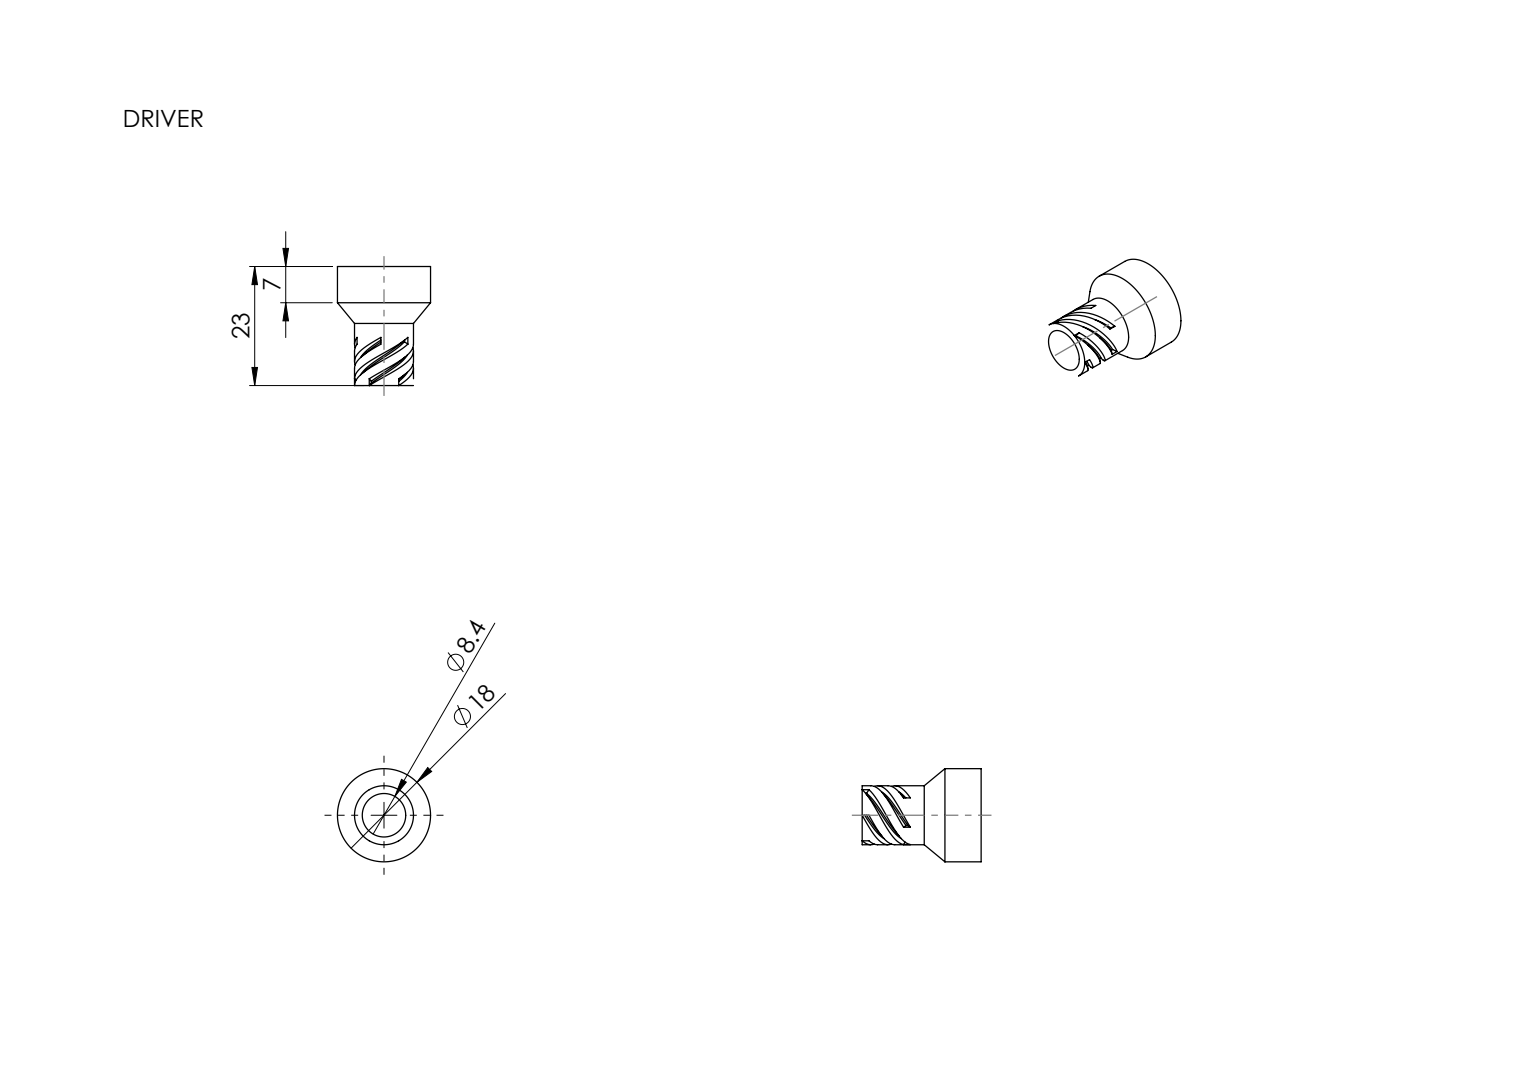
ISO-10303-21;
HEADER;
FILE_DESCRIPTION (('STEP AP214'),
    '1' );
FILE_NAME ('DRIVER.step',
    '2026-10-08T05:56:58',
    ( '' ),
    ( '' ),
    'SwSTEP 2.0',
    'SolidWorks 2026',
    '' );
FILE_SCHEMA (( 'AUTOMOTIVE_DESIGN' ));
ENDSEC;

DATA;
#10=ORIENTED_EDGE ( 'NONE', *, *, #9147, .T. ) ;
#12=CARTESIAN_POINT ( 'NONE',  ( 1.510506337161861223, 4.648860486681953397, -12.84374999795161543 ) ) ;
#32=( BOUNDED_CURVE ( )  B_SPLINE_CURVE ( 2, ( #2369, #8482, #14588, #875, #19172, #5461, #16578, #8772, #11868, #7343, #19367, #11771, #17980, #5752, #6052 ),
 .UNSPECIFIED., .F., .F. ) 
 B_SPLINE_CURVE_WITH_KNOTS ( ( 3, 2, 2, 2, 2, 2, 2, 3 ),
 ( 0.000000000000000000, 0.05000000000000000278, 0.1000000000000000056, 0.1499999999999999944, 0.2000000000000000111, 0.2500000000000000000, 0.2999999999999999889, 0.3333180920165871863 ),
 .UNSPECIFIED. ) 
 CURVE ( )  GEOMETRIC_REPRESENTATION_ITEM ( )  RATIONAL_B_SPLINE_CURVE ( ( 1.000000000000000000, 0.9876883405951377704, 1.000000000000000000, 0.9876883405951377704, 1.000000000000000000, 0.9876883405951377704, 1.000000000000000000, 0.9876883405951377704, 1.000000000000000000, 0.9876883405951377704, 1.000000000000000000, 0.9876883405951377704, 1.000000000000000000, 0.9917959799814384247, 0.9945256517182510247 ) ) 
 REPRESENTATION_ITEM ( '' )  );
#37=CARTESIAN_POINT ( 'NONE',  ( -5.207209108562804722, 2.318398865532109276, -15.31249999590322552 ) ) ;
#50=CARTESIAN_POINT ( 'NONE',  ( -1.493657965219562511, -5.574407415329147852, -9.812499995903225525 ) ) ;
#51=EDGE_CURVE ( 'NONE', #4769, #2089, #9336, .T. ) ;
#83=CARTESIAN_POINT ( 'NONE',  ( -4.620319390059805187, 1.773574444220790136, -11.34374999795161543 ) ) ;
#115=ORIENTED_EDGE ( 'NONE', *, *, #15621, .F. ) ;
#134=EDGE_CURVE ( 'NONE', #16351, #5756, #19323, .T. ) ;
#154=CARTESIAN_POINT ( 'NONE',  ( -5.700000000000001066, -0.5990941410143296730, -13.64430100820692537 ) ) ;
#159=CARTESIAN_POINT ( 'NONE',  ( 4.465502636338025688, -1.988169868018592412, -14.84374999795161543 ) ) ;
#163=EDGE_CURVE ( 'NONE', #5395, #4220, #13751, .T. ) ;
#168=FACE_OUTER_BOUND ( 'NONE', #5426, .T. ) ;
#169=CARTESIAN_POINT ( 'NONE',  ( 5.421022142882364392, -1.761396867937238486, -8.312499995903225525 ) ) ;
#180=CARTESIAN_POINT ( 'NONE',  ( -5.387740456496247887, -2.068159791354146293, -12.81249999590322552 ) ) ;
#184=CARTESIAN_POINT ( 'NONE',  ( 2.246813503491833508, 4.409619785863906571, -12.96874999795161543 ) ) ;
#214=CARTESIAN_POINT ( 'NONE',  ( 3.954556930911861112, 2.873153789725825913, -14.84374999795161543 ) ) ;
#216=EDGE_CURVE ( 'NONE', #1617, #5986, #4540, .T. ) ;
#221=CARTESIAN_POINT ( 'NONE',  ( -4.888101187500000222, 0.7741991708318887166, -6.968749997951614539 ) ) ;
#230=CARTESIAN_POINT ( 'NONE',  ( -3.270778111535363131, -3.632567103900500971, -10.84374999795161543 ) ) ;
#231=CARTESIAN_POINT ( 'NONE',  ( 2.444050593750020095, 4.233219804643871598, -6.468749997951615427 ) ) ;
#232=CARTESIAN_POINT ( 'NONE',  ( 4.942249507334556036, -0.2590123213421313686, -9.968749997951617203 ) ) ;
#234=CARTESIAN_POINT ( 'NONE',  ( 4.200000000000000178, 0.000000000000000000, -28.99999999999999645 ) ) ;
#256=CARTESIAN_POINT ( 'NONE',  ( 2.318398865532073749, 5.207209108562820710, -10.31249999590322552 ) ) ;
#266=EDGE_LOOP ( 'NONE', ( #427, #17181, #9017, #11698, #10341, #16603 ) ) ;
#270=EDGE_LOOP ( 'NONE', ( #16817, #14274, #8811, #901, #1434 ) ) ;
#274=CARTESIAN_POINT ( 'NONE',  ( -4.936344801571327601, -2.849999999999954792, -12.31249999590322552 ) ) ;
#275=CARTESIAN_POINT ( 'NONE',  ( -5.668774803599153422, 0.5958122406256767256, -13.00000000000000533 ) ) ;
#278=CARTESIAN_POINT ( 'NONE',  ( -4.409619785863906571, 2.246813503491833508, -7.968749997951616315 ) ) ;
#306=CARTESIAN_POINT ( 'NONE',  ( -2.246813503491833508, 4.409619785863906571, -10.34374999795161543 ) ) ;
#328=CARTESIAN_POINT ( 'NONE',  ( 4.465502636338039011, 1.988169868018562436, -8.468749997951615427 ) ) ;
#329=CARTESIAN_POINT ( 'NONE',  ( 4.780397808154266848, 1.280903732194421218, -8.968749997951611874 ) ) ;
#334=VECTOR ( 'NONE', #14992, 1000.000000000000000 ) ;
#347=ORIENTED_EDGE ( 'NONE', *, *, #1908, .F. ) ;
#353=EDGE_CURVE ( 'NONE', #3827, #6550, #12668, .T. ) ;
#354=CARTESIAN_POINT ( 'NONE',  ( -3.270778111535288080, 3.632567103900569361, -12.84374999795161543 ) ) ;
#356=AXIS2_PLACEMENT_3D ( 'NONE', #1344, #12254, #12353 ) ;
#369=CARTESIAN_POINT ( 'NONE',  ( 0.3020334839682081163, -5.763142191869158992, -8.812499995903225525 ) ) ;
#373=CARTESIAN_POINT ( 'NONE',  ( -4.611396867937201272, 3.350375938067097437, -8.000000000000005329 ) ) ;
#386=CARTESIAN_POINT ( 'NONE',  ( 5.668774803599163192, 0.5958122406255991210, -9.000000000000005329 ) ) ;
#427=ORIENTED_EDGE ( 'NONE', *, *, #9117, .T. ) ;
#431=CARTESIAN_POINT ( 'NONE',  ( 4.447186883680864788, 3.231070400981779667, -14.11718749948790830 ) ) ;
#434=CARTESIAN_POINT ( 'NONE',  ( 4.620319390059819398, -1.773574444220757274, -10.96874999795161720 ) ) ;
#443=EDGE_CURVE ( 'NONE', #4220, #16711, #7630, .T. ) ;
#446=ORIENTED_EDGE ( 'NONE', *, *, #14016, .F. ) ;
#476=ADVANCED_FACE ( 'NONE', ( #8445 ), #15472, .T. ) ;
#480=CARTESIAN_POINT ( 'NONE',  ( -3.143139765844555900, 4.840010801796527318, -12.50000000000000533 ) ) ;
#488=VERTEX_POINT ( 'NONE', #13041 ) ;
#500=SURFACE_SIDE_STYLE ('',( #17201 ) ) ;
#502=DIRECTION ( 'NONE',  ( -0.000000000000000000, -0.000000000000000000, 1.000000000000000000 ) ) ;
#513=CARTESIAN_POINT ( 'NONE',  ( 5.668774803599156975, -0.5958122406256373127, -14.31249999590322552 ) ) ;
#529=CARTESIAN_POINT ( 'NONE',  ( -9.000000000000001776, 0.000000000000000000, -22.00000000000000000 ) ) ;
#532=CARTESIAN_POINT ( 'NONE',  ( 5.700000000000001954, -0.5990941410143687529, -10.98069898359950258 ) ) ;
#535=DIRECTION ( 'NONE',  ( 1.000000000000000000, 0.000000000000000000, 0.000000000000000000 ) ) ;
#537=CARTESIAN_POINT ( 'NONE',  ( -4.942249507334558700, -0.2590123213420631454, -13.34374999795161365 ) ) ;
#544=EDGE_LOOP ( 'NONE', ( #8721, #12859, #15196, #3818, #16637 ) ) ;
#571=CARTESIAN_POINT ( 'NONE',  ( -2.318398865532109721, -5.207209108562803834, -9.000000000000005329 ) ) ;
#575=ORIENTED_EDGE ( 'NONE', *, *, #10908, .T. ) ;
#595=CARTESIAN_POINT ( 'NONE',  ( -1.510506337161893642, -4.648860486681943627, -12.46874999795161543 ) ) ;
#598=CARTESIAN_POINT ( 'NONE',  ( 0.000000000000000000, 0.000000000000000000, -28.99999999999999645 ) ) ;
#604=CARTESIAN_POINT ( 'NONE',  ( 3.270778111535314281, -3.632567103900546712, -12.84374999795161543 ) ) ;
#615=EDGE_CURVE ( 'NONE', #13431, #17330, #7505, .T. ) ;
#631=EDGE_CURVE ( 'NONE', #9247, #8012, #19426, .T. ) ;
#634=CARTESIAN_POINT ( 'NONE',  ( 3.632567103900546712, 3.270778111535313837, -7.843749997951614539 ) ) ;
#645=CIRCLE ( 'NONE', #13735, 5.700000000000002842 ) ;
#647=CARTESIAN_POINT ( 'NONE',  ( 2.246813503491803310, -4.409619785863921670, -9.968749997951615427 ) ) ;
#652=EDGE_LOOP ( 'NONE', ( #11686, #13562, #787, #7989 ) ) ;
#678=CARTESIAN_POINT ( 'NONE',  ( -1.493657965219446382, 5.574407415329178939, -13.50000000000000533 ) ) ;
#684=( BOUNDED_CURVE ( )  B_SPLINE_CURVE ( 2, ( #2775, #16596, #17896, #2575, #14700, #16400, #18096, #2876, #8691, #8990, #898, #990, #7068, #11693, #17798, #4094, #14800 ),
 .UNSPECIFIED., .F., .F. ) 
 B_SPLINE_CURVE_WITH_KNOTS ( ( 3, 2, 2, 2, 2, 2, 2, 2, 3 ),
 ( 0.000000000000000000, 0.05000000000000000971, 0.1000000000000000194, 0.1499999999999999944, 0.2000000000000000389, 0.2500000000000000000, 0.2999999999999999889, 0.3499999999999999223, 0.4000000000000000777 ),
 .UNSPECIFIED. ) 
 CURVE ( )  GEOMETRIC_REPRESENTATION_ITEM ( )  RATIONAL_B_SPLINE_CURVE ( ( 1.000000000000000000, 0.9876883405951377704, 1.000000000000000000, 0.9876883405951377704, 1.000000000000000000, 0.9876883405951377704, 1.000000000000000000, 0.9876883405951377704, 1.000000000000000000, 0.9876883405951377704, 1.000000000000000000, 0.9876883405951377704, 1.000000000000000000, 0.9876883405951377704, 1.000000000000000000, 0.9876883405951377704, 1.000000000000000000 ) ) 
 REPRESENTATION_ITEM ( '' )  );
#693=CARTESIAN_POINT ( 'NONE',  ( 5.142044285764733935, -2.620002426024580000, -7.500000000000005329 ) ) ;
#700=VECTOR ( 'NONE', #12818, 1000.000000000000000 ) ;
#707=CARTESIAN_POINT ( 'NONE',  ( 3.954556930911861112, 2.873153789725825913, -14.84374999795161543 ) ) ;
#732=CARTESIAN_POINT ( 'NONE',  ( 4.611396867937200383, 3.350375938067097881, -15.31249999590322552 ) ) ;
#736=VERTEX_POINT ( 'NONE', #10923 ) ;
#745=CARTESIAN_POINT ( 'NONE',  ( 5.421022142882364392, -1.761396867937238486, -8.312499995903225525 ) ) ;
#757=CARTESIAN_POINT ( 'NONE',  ( 0.000000000000000000, 0.000000000000000000, -28.99999999999999645 ) ) ;
#760=B_SPLINE_CURVE_WITH_KNOTS ( 'NONE', 1,
 ( #6972, #5479 ),
 .UNSPECIFIED., .F., .F.,
 ( 2, 2 ),
 ( 0.000000000000000000, 1.000000000000000000 ),
 .UNSPECIFIED. ) ;
#768=VERTEX_POINT ( 'NONE', #1106 ) ;
#772=CARTESIAN_POINT ( 'NONE',  ( -4.780397808154273953, -1.280903732194386579, -8.968749997951611874 ) ) ;
#778=FACE_OUTER_BOUND ( 'NONE', #6078, .T. ) ;
#782=ORIENTED_EDGE ( 'NONE', *, *, #15988, .T. ) ;
#787=ORIENTED_EDGE ( 'NONE', *, *, #9672, .F. ) ;
#790=EDGE_CURVE ( 'NONE', #17079, #15015, #15922, .T. ) ;
#798=ORIENTED_EDGE ( 'NONE', *, *, #9859, .T. ) ;
#803=CARTESIAN_POINT ( 'NONE',  ( 1.493657965219485462, -5.574407415329169169, -14.81249999590322552 ) ) ;
#805=( BOUNDED_SURFACE ( )  B_SPLINE_SURFACE ( 1, 2, ( 
 ( #16231, #11437, #17538, #3824, #17827, #9121, #4217, #4316, #13231, #11820, #13517, #19717, #19317, #10427, #6000, #15122, #10232 ),
 ( #4119, #11722, #1314, #10524, #14925, #17927, #8719, #5609, #2806, #16728, #14826, #16326, #16528, #5906, #13620, #3008, #12123 ) ),
 .UNSPECIFIED., .F., .F., .F. ) 
 B_SPLINE_SURFACE_WITH_KNOTS ( ( 2, 2 ),
 ( 3, 2, 2, 2, 2, 2, 2, 2, 3 ),
 ( 0.000000000000000000, 1.000000000000000000 ),
 ( 0.000000000000000000, 0.05000000000000000278, 0.1000000000000000056, 0.1499999999999999944, 0.2000000000000000111, 0.2500000000000000000, 0.2999999999999999889, 0.3499999999999999778, 0.4000000000000000222 ),
 .UNSPECIFIED. ) 
 GEOMETRIC_REPRESENTATION_ITEM ( )  RATIONAL_B_SPLINE_SURFACE ( (
 ( 1.000000000000000000, 0.9876883405951377704, 1.000000000000000000, 0.9876883405951377704, 1.000000000000000000, 0.9876883405951377704, 1.000000000000000000, 0.9876883405951377704, 1.000000000000000000, 0.9876883405951377704, 1.000000000000000000, 0.9876883405951377704, 1.000000000000000000, 0.9876883405951377704, 1.000000000000000000, 0.9876883405951377704, 1.000000000000000000),
 ( 1.000000000000000000, 0.9876883405951377704, 1.000000000000000000, 0.9876883405951377704, 1.000000000000000000, 0.9876883405951377704, 1.000000000000000000, 0.9876883405951377704, 1.000000000000000000, 0.9876883405951377704, 1.000000000000000000, 0.9876883405951377704, 1.000000000000000000, 0.9876883405951377704, 1.000000000000000000, 0.9876883405951377704, 1.000000000000000000) ) ) 
 REPRESENTATION_ITEM ( '' )  SURFACE ( )  );
#838=EDGE_CURVE ( 'NONE', #8012, #12976, #9469, .T. ) ;
#842=CARTESIAN_POINT ( 'NONE',  ( 1.510506337161829027, -4.648860486681964055, -10.84374999795161543 ) ) ;
#847=VECTOR ( 'NONE', #4218, 1000.000000000000000 ) ;
#859=AXIS2_PLACEMENT_3D ( 'NONE', #9005, #17910, #4106 ) ;
#868=CARTESIAN_POINT ( 'NONE',  ( 4.861323657744406113, -0.5109457054261780096, -13.46874999795161543 ) ) ;
#875=CARTESIAN_POINT ( 'NONE',  ( -0.3020334839682475847, 5.763142191869157216, -7.500000000000005329 ) ) ;
#880=VECTOR ( 'NONE', #12534, 1000.000000000000000 ) ;
#896=CARTESIAN_POINT ( 'NONE',  ( 3.814044456245474279, -4.235925505221167064, -13.31249999590322730 ) ) ;
#898=CARTESIAN_POINT ( 'NONE',  ( 4.233219804643871598, -2.444050593750019651, -11.46874999795161543 ) ) ;
#901=ORIENTED_EDGE ( 'NONE', *, *, #9677, .T. ) ;
#903=CARTESIAN_POINT ( 'NONE',  ( -9.000000000000001776, 1.102182119232617911E-15, -22.00000000000000000 ) ) ;
#906=DIRECTION ( 'NONE',  ( 1.000000000000000000, 0.000000000000000000, 0.000000000000000000 ) ) ;
#909=CARTESIAN_POINT ( 'NONE',  ( -2.647025296874989664, 4.584782303107598267, -6.234374998975811266 ) ) ;
#915=DIRECTION ( 'NONE',  ( -0.000000000000000000, -0.000000000000000000, 1.000000000000000000 ) ) ;
#924=VECTOR ( 'NONE', #15469, 1000.000000000000000 ) ;
#947=CARTESIAN_POINT ( 'NONE',  ( -2.873153789725852558, -3.954556930911842016, -13.46874999795161543 ) ) ;
#958=CARTESIAN_POINT ( 'NONE',  ( -3.114526743279308896, -3.846120219227901149, -7.343749997951615427 ) ) ;
#959=FACE_OUTER_BOUND ( 'NONE', #270, .T. ) ;
#980=FACE_OUTER_BOUND ( 'NONE', #5717, .T. ) ;
#988=CARTESIAN_POINT ( 'NONE',  ( 4.465502636338039011, 1.988169868018562436, -8.843749997951615427 ) ) ;
#990=CARTESIAN_POINT ( 'NONE',  ( 3.846120219227923798, -3.114526743279282250, -11.96874999795161365 ) ) ;
#992=CARTESIAN_POINT ( 'NONE',  ( -3.270778111535363131, -3.632567103900500971, -10.84374999795161543 ) ) ;
#995=CARTESIAN_POINT ( 'NONE',  ( 4.235925505221166176, 3.814044456245473835, -8.312499995903225525 ) ) ;
#1012=CARTESIAN_POINT ( 'NONE',  ( -3.350375938067097437, 4.611396867937201272, -9.000000000000005329 ) ) ;
#1016=AXIS2_PLACEMENT_3D ( 'NONE', #3831, #10049, #2613 ) ;
#1022=CARTESIAN_POINT ( 'NONE',  ( -0.5958122406255597081, 5.668774803599165857, -14.00000000000000533 ) ) ;
#1025=CARTESIAN_POINT ( 'NONE',  ( 2.850000000000024070, 4.936344801571289409, -6.000000000000005329 ) ) ;
#1026=CARTESIAN_POINT ( 'NONE',  ( 5.699999596629369059, -0.002144393866035136480, -6.000593838912648081 ) ) ;
#1050=ORIENTED_EDGE ( 'NONE', *, *, #3700, .F. ) ;
#1059=CARTESIAN_POINT ( 'NONE',  ( -4.233219804643852946, 2.444050593750049405, -11.84374999795161365 ) ) ;
#1061=CARTESIAN_POINT ( 'NONE',  ( 2.695436003842732298, 4.150607464521791634, -9.968749997951617203 ) ) ;
#1063=ORIENTED_EDGE ( 'NONE', *, *, #9677, .F. ) ;
#1073=B_SPLINE_CURVE_WITH_KNOTS ( 'NONE', 1,
 ( #8978, #2969 ),
 .UNSPECIFIED., .F., .F.,
 ( 2, 2 ),
 ( 0.000000000000000000, 1.000000000000000000 ),
 .UNSPECIFIED. ) ;
#1093=CARTESIAN_POINT ( 'NONE',  ( -4.080749450109650844, 4.080749450109650844, -9.812499995903223748 ) ) ;
#1099=EDGE_LOOP ( 'NONE', ( #1954, #16438, #575, #16915 ) ) ;
#1103=EDGE_CURVE ( 'NONE', #13293, #13685, #7982, .T. ) ;
#1106=CARTESIAN_POINT ( 'NONE',  ( -5.700000000000002842, 0.000000000000000000, -18.00000000000000355 ) ) ;
#1119=CARTESIAN_POINT ( 'NONE',  ( 4.611396867937200383, 3.350375938067097881, -14.00000000000000533 ) ) ;
#1130=CARTESIAN_POINT ( 'NONE',  ( 4.840010801796506001, 3.143139765844590983, -7.500000000000005329 ) ) ;
#1144=CARTESIAN_POINT ( 'NONE',  ( -3.954556930911881096, -2.873153789725797935, -14.46874999795161720 ) ) ;
#1146=CARTESIAN_POINT ( 'NONE',  ( -4.465502636338010589, 1.988169868018623720, -14.84374999795161543 ) ) ;
#1147=EDGE_LOOP ( 'NONE', ( #4096, #3789, #12811, #6049 ) ) ;
#1153=ORIENTED_EDGE ( 'NONE', *, *, #6590, .T. ) ;
#1156=CARTESIAN_POINT ( 'NONE',  ( 0.000000000000000000, 0.000000000000000000, -6.000000000000005329 ) ) ;
#1158=CARTESIAN_POINT ( 'NONE',  ( 4.465502636338025688, -1.988169868018592856, -14.46874999795161720 ) ) ;
#1160=CARTESIAN_POINT ( 'NONE',  ( 0.5958122406256377568, 5.668774803599156975, -9.312499995903225525 ) ) ;
#1195=CARTESIAN_POINT ( 'NONE',  ( 0.5958122406255995651, -5.668774803599162304, -14.00000000000000533 ) ) ;
#1196=EDGE_LOOP ( 'NONE', ( #11214, #10475, #18129, #3079 ) ) ;
#1206=CARTESIAN_POINT ( 'NONE',  ( 4.888101187500000222, -3.413342815706642518E-14, -6.468749997951615427 ) ) ;
#1224=CARTESIAN_POINT ( 'NONE',  ( 4.620319390059829168, 1.773574444220725299, -11.96874999795161365 ) ) ;
#1235=CARTESIAN_POINT ( 'NONE',  ( -3.499494075959840078, -3.499494075959791672, -14.34374999795161365 ) ) ;
#1256=CARTESIAN_POINT ( 'NONE',  ( -0.3020334839682475847, 5.763142191869157216, -7.500000000000005329 ) ) ;
#1288=CARTESIAN_POINT ( 'NONE',  ( -4.840010801796527318, -3.143139765844555900, -8.812499995903225525 ) ) ;
#1291=CARTESIAN_POINT ( 'NONE',  ( -4.942249507334554259, 0.2590123213421660631, -9.968749997951615427 ) ) ;
#1308=FACE_OUTER_BOUND ( 'NONE', #10180, .T. ) ;
#1314=CARTESIAN_POINT ( 'NONE',  ( 1.016293382781377819, -4.781284448697200595, -7.468749997951615427 ) ) ;
#1320=CARTESIAN_POINT ( 'NONE',  ( -3.499494075959840078, -3.499494075959792116, -14.34374999795161543 ) ) ;
#1322=CARTESIAN_POINT ( 'NONE',  ( -0.2590123213420971182, 4.942249507334556924, -7.968749997951616315 ) ) ;
#1343=ORIENTED_EDGE ( 'NONE', *, *, #8950, .F. ) ;
#1344=CARTESIAN_POINT ( 'NONE',  ( 2.647025296875021638, 4.584782303107579615, -6.234374998975811266 ) ) ;
#1346=VERTEX_POINT ( 'NONE', #4276 ) ;
#1349=VECTOR ( 'NONE', #9495, 1000.000000000000000 ) ;
#1350=CARTESIAN_POINT ( 'NONE',  ( 1.988169868018562880, -4.465502636338038123, -13.46874999795161543 ) ) ;
#1358=CARTESIAN_POINT ( 'NONE',  ( 5.207209108562820710, -2.318398865532073305, -14.00000000000000533 ) ) ;
#1384=ORIENTED_EDGE ( 'NONE', *, *, #5542, .T. ) ;
#1389=CARTESIAN_POINT ( 'NONE',  ( -5.700000000000000178, 0.5990941410143899581, -9.668198987696271729 ) ) ;
#1392=CARTESIAN_POINT ( 'NONE',  ( 4.465502636338025688, -1.988169868018592412, -14.84374999795161543 ) ) ;
#1393=CARTESIAN_POINT ( 'NONE',  ( -5.387740456496206143, 2.068159791354259092, -11.81249999590322552 ) ) ;
#1396=CARTESIAN_POINT ( 'NONE',  ( -4.233219804643852946, 2.444050593750049405, -11.46874999795161543 ) ) ;
#1422=AXIS2_PLACEMENT_3D ( 'NONE', #9159, #13556, #15159 ) ;
#1423=CARTESIAN_POINT ( 'NONE',  ( -2.647025296874989664, 4.584782303107598267, -7.078124996927420476 ) ) ;
#1426=CARTESIAN_POINT ( 'NONE',  ( 4.233219804643887585, 2.444050593749990785, -11.46874999795161543 ) ) ;
#1434=ORIENTED_EDGE ( 'NONE', *, *, #14888, .F. ) ;
#1458=CARTESIAN_POINT ( 'NONE',  ( 4.484949146646379781, 3.631840208645794821, -10.50000000000000711 ) ) ;
#1462=VERTEX_POINT ( 'NONE', #14451 ) ;
#1474=CARTESIAN_POINT ( 'NONE',  ( 1.761396867937162769, -5.421022142882388373, -11.31249999590322375 ) ) ;
#1487=CARTESIAN_POINT ( 'NONE',  ( 0.7741991708318884946, 4.888101187500000222, -12.34374999795161543 ) ) ;
#1504=CARTESIAN_POINT ( 'NONE',  ( 1.988169868018562880, -4.465502636338038123, -13.84374999795161543 ) ) ;
#1514=VERTEX_POINT ( 'NONE', #9958 ) ;
#1524=CARTESIAN_POINT ( 'NONE',  ( -3.954556930911862000, 2.873153789725825469, -8.468749997951615427 ) ) ;
#1532=CARTESIAN_POINT ( 'NONE',  ( 5.294050593750000644, -3.696815770993907903E-14, -6.234374998975811266 ) ) ;
#1536=CARTESIAN_POINT ( 'NONE',  ( -5.668774803599165857, -0.5958122406255588199, -9.000000000000005329 ) ) ;
#1550=CARTESIAN_POINT ( 'NONE',  ( 2.850000000000024070, 4.936344801571289409, -6.000000000000005329 ) ) ;
#1554=CARTESIAN_POINT ( 'NONE',  ( -5.763142191869158992, -0.3020334839682081163, -12.50000000000000533 ) ) ;
#1556=ORIENTED_EDGE ( 'NONE', *, *, #8950, .T. ) ;
#1557=( BOUNDED_CURVE ( )  B_SPLINE_CURVE ( 2, ( #1026, #14552, #14649, #11354, #13044, #18945, #11448, #13241, #2522, #8631, #5527, #5429, #7110, #19233, #19328, #8541, #5235 ),
 .UNSPECIFIED., .F., .F. ) 
 B_SPLINE_CURVE_WITH_KNOTS ( ( 3, 2, 2, 2, 2, 2, 2, 2, 3 ),
 ( 0.000000000000000000, 0.05000000000000000971, 0.1000000000000000194, 0.1499999999999999944, 0.2000000000000000389, 0.2500000000000000000, 0.2999999999999999889, 0.3499999999999999223, 0.4000000000000000777 ),
 .UNSPECIFIED. ) 
 CURVE ( )  GEOMETRIC_REPRESENTATION_ITEM ( )  RATIONAL_B_SPLINE_CURVE ( ( 1.000000000000000000, 0.9876883405951377704, 1.000000000000000000, 0.9876883405951377704, 1.000000000000000000, 0.9876883405951377704, 1.000000000000000000, 0.9876883405951377704, 1.000000000000000000, 0.9876883405951377704, 1.000000000000000000, 0.9876883405951377704, 1.000000000000000000, 0.9876883405951377704, 1.000000000000000000, 0.9876883405951377704, 1.000000000000000000 ) ) 
 REPRESENTATION_ITEM ( '' )  );
#1609=VECTOR ( 'NONE', #17718, 1000.000000000000000 ) ;
#1615=CARTESIAN_POINT ( 'NONE',  ( -3.954556930911862000, 2.873153789725825469, -8.843749997951615427 ) ) ;
#1617=VERTEX_POINT ( 'NONE', #13630 ) ;
#1633=ORIENTED_EDGE ( 'NONE', *, *, #14674, .F. ) ;
#1653=CARTESIAN_POINT ( 'NONE',  ( -5.387740456496247887, -2.068159791354146293, -11.50000000000000355 ) ) ;
#1654=CARTESIAN_POINT ( 'NONE',  ( -5.700000000000000178, -2.180340287075187351E-16, -13.97977757194593273 ) ) ;
#1660=EDGE_CURVE ( 'NONE', #5242, #16351, #10502, .T. ) ;
#1670=( BOUNDED_CURVE ( )  B_SPLINE_CURVE ( 2, ( #7922, #19032, #5323, #12936, #2509, #11720, #1012, #17925, #7193, #4117, #6811, #19128, #8717, #14824, #17727, #7095, #1119 ),
 .UNSPECIFIED., .F., .F. ) 
 B_SPLINE_CURVE_WITH_KNOTS ( ( 3, 2, 2, 2, 2, 2, 2, 2, 3 ),
 ( 0.000000000000000000, 0.05000000000000000971, 0.1000000000000000194, 0.1499999999999999944, 0.2000000000000000389, 0.2500000000000000000, 0.2999999999999999889, 0.3499999999999999223, 0.4000000000000000777 ),
 .UNSPECIFIED. ) 
 CURVE ( )  GEOMETRIC_REPRESENTATION_ITEM ( )  RATIONAL_B_SPLINE_CURVE ( ( 1.000000000000000000, 0.9876883405951377704, 1.000000000000000000, 0.9876883405951377704, 1.000000000000000000, 0.9876883405951377704, 1.000000000000000000, 0.9876883405951377704, 1.000000000000000000, 0.9876883405951377704, 1.000000000000000000, 0.9876883405951377704, 1.000000000000000000, 0.9876883405951377704, 1.000000000000000000, 0.9876883405951377704, 1.000000000000000000 ) ) 
 REPRESENTATION_ITEM ( '' )  );
#1686=CARTESIAN_POINT ( 'NONE',  ( -1.988169868018530906, 4.465502636338051445, -13.84374999795161543 ) ) ;
#1692=DIRECTION ( 'NONE',  ( 0.4330127018922284576, 0.7499999999999961142, 0.4999999999999977240 ) ) ;
#1696=CARTESIAN_POINT ( 'NONE',  ( -5.668774803599165857, -0.5958122406255588199, -10.31249999590322552 ) ) ;
#1708=CARTESIAN_POINT ( 'NONE',  ( 1.493657965219485462, -5.574407415329169169, -13.50000000000000533 ) ) ;
#1714=CARTESIAN_POINT ( 'NONE',  ( -3.954556930911862000, 2.873153789725825469, -8.843749997951615427 ) ) ;
#1759=CARTESIAN_POINT ( 'NONE',  ( 5.763142191869157216, 0.3020334839682480288, -13.81249999590322552 ) ) ;
#1779=CARTESIAN_POINT ( 'NONE',  ( -1.761396867937200739, 5.421022142882375938, -10.00000000000000533 ) ) ;
#1791=CARTESIAN_POINT ( 'NONE',  ( -4.611396867937224364, -3.350375938067065906, -14.00000000000000533 ) ) ;
#1794=( NAMED_UNIT ( * ) SI_UNIT ( $, .STERADIAN. ) SOLID_ANGLE_UNIT ( ) );
#1808=EDGE_LOOP ( 'NONE', ( #15620, #13680, #16181, #1384 ) ) ;
#1810=FACE_OUTER_BOUND ( 'NONE', #1196, .T. ) ;
#1816=AXIS2_PLACEMENT_3D ( 'NONE', #1532, #10443, #7619 ) ;
#1820=VECTOR ( 'NONE', #5810, 1000.000000000000000 ) ;
#1821=ORIENTED_EDGE ( 'NONE', *, *, #10236, .T. ) ;
#1824=CARTESIAN_POINT ( 'NONE',  ( 5.700000000000002842, 2.725425358843983450E-16, -10.64522241986047568 ) ) ;
#1874=CARTESIAN_POINT ( 'NONE',  ( -3.143139765844656708, -4.840010801796461593, -10.81249999590322375 ) ) ;
#1877=CARTESIAN_POINT ( 'NONE',  ( -2.246813503491833508, 4.409619785863906571, -9.968749997951617203 ) ) ;
#1883=CARTESIAN_POINT ( 'NONE',  ( -2.647025296875054057, -4.584782303107560963, -7.078124996927420476 ) ) ;
#1888=CARTESIAN_POINT ( 'NONE',  ( -3.631840208645857437, -4.484949146646330931, -7.812499995903224637 ) ) ;
#1894=DIRECTION ( 'NONE',  ( 1.000000000000000000, 0.000000000000000000, 0.000000000000000000 ) ) ;
#1899=VERTEX_POINT ( 'NONE', #6993 ) ;
#1908=EDGE_CURVE ( 'NONE', #7839, #10504, #16759, .T. ) ;
#1914=ORIENTED_EDGE ( 'NONE', *, *, #9622, .T. ) ;
#1925=CARTESIAN_POINT ( 'NONE',  ( 4.861323657744411442, 0.5109457054261445919, -9.468749997951615427 ) ) ;
#1941=SHAPE_DEFINITION_REPRESENTATION ( #10190, #6040 ) ;
#1942=CARTESIAN_POINT ( 'NONE',  ( -3.143139765844656708, -4.840010801796461593, -9.500000000000003553 ) ) ;
#1954=ORIENTED_EDGE ( 'NONE', *, *, #9226, .T. ) ;
#1959=CARTESIAN_POINT ( 'NONE',  ( -5.387740456496247887, -2.068159791354146293, -11.50000000000000355 ) ) ;
#1971=CARTESIAN_POINT ( 'NONE',  ( -2.318398865532001363, 5.207209108562852684, -14.31249999590322552 ) ) ;
#1978=CARTESIAN_POINT ( 'NONE',  ( 5.207209108562820710, -2.318398865532073305, -14.00000000000000533 ) ) ;
#1985=CARTESIAN_POINT ( 'NONE',  ( -3.499494075959840078, -3.499494075959791672, -13.96874999795161365 ) ) ;
#1989=LINE ( 'NONE', #13905, #16458 ) ;
#1996=CARTESIAN_POINT ( 'NONE',  ( 5.700000000000002842, 2.725425358843983450E-16, -9.332722423957255486 ) ) ;
#2001=CARTESIAN_POINT ( 'NONE',  ( 5.207209108562820710, -2.318398865532073305, -15.31249999590322552 ) ) ;
#2013=ORIENTED_EDGE ( 'NONE', *, *, #9226, .F. ) ;
#2027=CARTESIAN_POINT ( 'NONE',  ( 4.781284448697187273, -1.016293382781444654, -10.46874999795161720 ) ) ;
#2031=CARTESIAN_POINT ( 'NONE',  ( 5.207209108562820710, -2.318398865532073305, -15.31249999590322552 ) ) ;
#2053=CARTESIAN_POINT ( 'NONE',  ( -4.861323657744413218, -0.5109457054261099529, -9.843749997951615427 ) ) ;
#2066=ORIENTED_EDGE ( 'NONE', *, *, #4858, .T. ) ;
#2072=CARTESIAN_POINT ( 'NONE',  ( -4.080749450109650844, 4.080749450109650844, -8.500000000000007105 ) ) ;
#2082=EDGE_CURVE ( 'NONE', #3194, #17426, #1989, .T. ) ;
#2083=CARTESIAN_POINT ( 'NONE',  ( 3.499494075959791672, -3.499494075959840966, -8.968749997951611874 ) ) ;
#2086=PRESENTATION_STYLE_ASSIGNMENT (( #5182 ) ) ;
#2089=VERTEX_POINT ( 'NONE', #9508 ) ;
#2093=CARTESIAN_POINT ( 'NONE',  ( 5.387740456496221242, -2.068159791354221344, -11.81249999590322552 ) ) ;
#2112=CARTESIAN_POINT ( 'NONE',  ( -5.700000000000000178, 0.5990941410143899581, -10.98069898359949192 ) ) ;
#2139=PLANE ( 'NONE',  #10424 ) ;
#2142=DIRECTION ( 'NONE',  ( 0.4330127018922234616, 0.7499999999999990008, 0.4999999999999978351 ) ) ;
#2154=CARTESIAN_POINT ( 'NONE',  ( -4.620319390059805187, 1.773574444220789914, -11.34374999795161543 ) ) ;
#2156=VECTOR ( 'NONE', #12013, 1000.000000000000000 ) ;
#2176=ORIENTED_EDGE ( 'NONE', *, *, #16459, .F. ) ;
#2179=EDGE_CURVE ( 'NONE', #8042, #9505, #19555, .T. ) ;
#2182=CARTESIAN_POINT ( 'NONE',  ( 2.246813503491803310, -4.409619785863921670, -9.968749997951617203 ) ) ;
#2189=CARTESIAN_POINT ( 'NONE',  ( 4.942249507334556036, -0.2590123213421313686, -10.34374999795161543 ) ) ;
#2190=( BOUNDED_CURVE ( )  B_SPLINE_CURVE ( 2, ( #18415, #15020, #19618, #13717, #2804, #7497, #6098, #18321, #5904, #12219, #10816, #15224, #12022, #16829, #10425, #18124, #2702 ),
 .UNSPECIFIED., .F., .F. ) 
 B_SPLINE_CURVE_WITH_KNOTS ( ( 3, 2, 2, 2, 2, 2, 2, 2, 3 ),
 ( 0.000000000000000000, 0.05000000000000000971, 0.1000000000000000194, 0.1499999999999999944, 0.2000000000000000389, 0.2500000000000000000, 0.2999999999999999889, 0.3499999999999999223, 0.4000000000000000777 ),
 .UNSPECIFIED. ) 
 CURVE ( )  GEOMETRIC_REPRESENTATION_ITEM ( )  RATIONAL_B_SPLINE_CURVE ( ( 1.000000000000000000, 0.9876883405951377704, 1.000000000000000000, 0.9876883405951377704, 1.000000000000000000, 0.9876883405951377704, 1.000000000000000000, 0.9876883405951377704, 1.000000000000000000, 0.9876883405951377704, 1.000000000000000000, 0.9876883405951377704, 1.000000000000000000, 0.9876883405951377704, 1.000000000000000000, 0.9876883405951377704, 1.000000000000000000 ) ) 
 REPRESENTATION_ITEM ( '' )  );
#2193=CARTESIAN_POINT ( 'NONE',  ( -2.873153789725825469, 3.954556930911862000, -9.843749997951615427 ) ) ;
#2194=EDGE_LOOP ( 'NONE', ( #16775, #7527, #12166, #10500 ) ) ;
#2196=ADVANCED_FACE ( 'NONE', ( #18598 ), #5183, .T. ) ;
#2201=FACE_OUTER_BOUND ( 'NONE', #18950, .T. ) ;
#2210=ORIENTED_EDGE ( 'NONE', *, *, #7191, .F. ) ;
#2218=CARTESIAN_POINT ( 'NONE',  ( 0.000000000000000000, 0.000000000000000000, -22.00000000000000000 ) ) ;
#2221=CARTESIAN_POINT ( 'NONE',  ( 3.632567103900546712, 3.270778111535313837, -7.468749997951615427 ) ) ;
#2222=ORIENTED_EDGE ( 'NONE', *, *, #15682, .F. ) ;
#2235=CARTESIAN_POINT ( 'NONE',  ( -1.510506337161893642, -4.648860486681943627, -12.46874999795161543 ) ) ;
#2261=EDGE_LOOP ( 'NONE', ( #7376, #6155, #6525, #11274, #6937 ) ) ;
#2317=CARTESIAN_POINT ( 'NONE',  ( 4.080749450109649956, 4.080749450109650844, -14.81249999590322375 ) ) ;
#2322=EDGE_CURVE ( 'NONE', #1899, #15854, #8394, .T. ) ;
#2330=CARTESIAN_POINT ( 'NONE',  ( 2.873153789725797491, -3.954556930911881985, -9.843749997951615427 ) ) ;
#2366=CARTESIAN_POINT ( 'NONE',  ( -4.611396867937224364, -3.350375938067065906, -15.31249999590322552 ) ) ;
#2369=CARTESIAN_POINT ( 'NONE',  ( -2.849999999999988987, 4.936344801571308061, -6.000000000000005329 ) ) ;
#2388=CARTESIAN_POINT ( 'NONE',  ( 3.632567103900546712, 3.270778111535313837, -7.843749997951614539 ) ) ;
#2391=CARTESIAN_POINT ( 'NONE',  ( 3.350375938067096548, 4.611396867937201272, -14.31249999590322552 ) ) ;
#2394=CARTESIAN_POINT ( 'NONE',  ( 5.207209108562838473, 2.318398865532038666, -9.312499995903225525 ) ) ;
#2400=FACE_OUTER_BOUND ( 'NONE', #5133, .T. ) ;
#2424=CARTESIAN_POINT ( 'NONE',  ( 0.5109457054261454800, -4.861323657744410554, -14.84374999795161543 ) ) ;
#2447=CARTESIAN_POINT ( 'NONE',  ( -4.942249507334553371, 0.2590123213421660631, -9.968749997951617203 ) ) ;
#2455=CARTESIAN_POINT ( 'NONE',  ( -4.781284448697179279, 1.016293382781477961, -10.46874999795161720 ) ) ;
#2478=CARTESIAN_POINT ( 'NONE',  ( 4.233219804643871598, -2.444050593750019651, -11.84374999795161365 ) ) ;
#2482=CARTESIAN_POINT ( 'NONE',  ( -0.9027913098498572264, 5.699999999999999289, -11.81249999590322552 ) ) ;
#2494=ORIENTED_EDGE ( 'NONE', *, *, #10561, .T. ) ;
#2496=CARTESIAN_POINT ( 'NONE',  ( 3.954556930911861112, 2.873153789725825913, -14.46874999795161720 ) ) ;
#2509=CARTESIAN_POINT ( 'NONE',  ( -4.611396867937201272, 3.350375938067097437, -8.000000000000005329 ) ) ;
#2517=CARTESIAN_POINT ( 'NONE',  ( -0.5109457054261112852, 4.861323657744413218, -14.46874999795161720 ) ) ;
#2522=CARTESIAN_POINT ( 'NONE',  ( 1.761396867937162769, -5.421022142882388373, -10.00000000000000533 ) ) ;
#2540=DIRECTION ( 'NONE',  ( 1.000000000000000000, 0.000000000000000000, 0.000000000000000000 ) ) ;
#2544=CARTESIAN_POINT ( 'NONE',  ( -2.444050593749990341, 4.233219804643887585, -6.468749997951615427 ) ) ;
#2574=CARTESIAN_POINT ( 'NONE',  ( -2.318398865532001363, 5.207209108562852684, -13.00000000000000533 ) ) ;
#2575=CARTESIAN_POINT ( 'NONE',  ( 4.150607464521811174, 2.695436003842704764, -7.968749997951616315 ) ) ;
#2577=CARTESIAN_POINT ( 'NONE',  ( 0.9027913098498566713, 5.699999999999999289, -12.81249999590322552 ) ) ;
#2582=CARTESIAN_POINT ( 'NONE',  ( 5.700000000000001954, 0.2987243419133224775, -10.47794484381774538 ) ) ;
#2597=VERTEX_POINT ( 'NONE', #12384 ) ;
#2603=CARTESIAN_POINT ( 'NONE',  ( -1.761396867937200739, 5.421022142882375938, -11.31249999590322375 ) ) ;
#2613=DIRECTION ( 'NONE',  ( 1.000000000000000000, 0.000000000000000000, 0.000000000000000000 ) ) ;
#2616=CARTESIAN_POINT ( 'NONE',  ( 1.280903732194454303, 4.780397808154257078, -8.968749997951611874 ) ) ;
#2642=DIRECTION ( 'NONE',  ( -0.000000000000000000, -0.000000000000000000, 1.000000000000000000 ) ) ;
#2643=VECTOR ( 'NONE', #18602, 1000.000000000000000 ) ;
#2645=VERTEX_POINT ( 'NONE', #8564 ) ;
#2658=VECTOR ( 'NONE', #17100, 1000.000000000000114 ) ;
#2672=LINE ( 'NONE', #8788, #16879 ) ;
#2674=CARTESIAN_POINT ( 'NONE',  ( -5.387740456496205255, 2.068159791354258648, -10.50000000000000533 ) ) ;
#2680=CARTESIAN_POINT ( 'NONE',  ( 5.668774803599163192, 0.5958122406255991210, -10.31249999590322552 ) ) ;
#2684=EDGE_CURVE ( 'NONE', #12845, #19252, #3862, .T. ) ;
#2692=CARTESIAN_POINT ( 'NONE',  ( 3.846120219227923798, -3.114526743279282250, -12.34374999795161543 ) ) ;
#2695=ADVANCED_FACE ( 'NONE', ( #959 ), #16118, .T. ) ;
#2702=CARTESIAN_POINT ( 'NONE',  ( 4.465502636338025688, -1.988169868018592412, -14.84374999795161543 ) ) ;
#2711=ADVANCED_FACE ( 'NONE', ( #7138 ), #14866, .F. ) ;
#2713=CARTESIAN_POINT ( 'NONE',  ( -3.383411828340740850E-14, -4.888101187500000222, -11.84374999795161365 ) ) ;
#2715=CARTESIAN_POINT ( 'NONE',  ( 0.5109457054261784537, 4.861323657744407001, -8.843749997951615427 ) ) ;
#2718=ORIENTED_EDGE ( 'NONE', *, *, #18316, .F. ) ;
#2740=CARTESIAN_POINT ( 'NONE',  ( 4.942249507334556036, -0.2590123213421313686, -9.968749997951617203 ) ) ;
#2746=CARTESIAN_POINT ( 'NONE',  ( 1.493657965219523875, 5.574407415329156734, -8.500000000000007105 ) ) ;
#2754=ADVANCED_FACE ( 'NONE', ( #16773 ), #12549, .T. ) ;
#2765=CARTESIAN_POINT ( 'NONE',  ( 5.142044285764733935, -2.620002426024580000, -8.812499995903225525 ) ) ;
#2768=DIRECTION ( 'NONE',  ( 1.000000000000000000, 0.000000000000000000, 0.000000000000000000 ) ) ;
#2774=LINE ( 'NONE', #8890, #334 ) ;
#2775=CARTESIAN_POINT ( 'NONE',  ( 2.444050593750020095, 4.233219804643871598, -6.468749997951615427 ) ) ;
#2781=CARTESIAN_POINT ( 'NONE',  ( -4.150607464521828938, -2.695436003842674122, -7.968749997951616315 ) ) ;
#2804=CARTESIAN_POINT ( 'NONE',  ( 0.5109457054261780096, 4.861323657744407001, -8.843749997951615427 ) ) ;
#2806=CARTESIAN_POINT ( 'NONE',  ( -3.270778111535363131, -3.632567103900500971, -10.46874999795161720 ) ) ;
#2811=CARTESIAN_POINT ( 'NONE',  ( -4.409619785863906571, 2.246813503491833508, -7.968749997951616315 ) ) ;
#2830=CARTESIAN_POINT ( 'NONE',  ( -3.954556930911881096, -2.873153789725797935, -14.84374999795161543 ) ) ;
#2831=( BOUNDED_CURVE ( )  B_SPLINE_CURVE ( 2, ( #15093, #1389, #4092, #2674, #7468, #7362, #16297, #4287, #2574, #7166, #19386 ),
 .UNSPECIFIED., .F., .F. ) 
 B_SPLINE_CURVE_WITH_KNOTS ( ( 3, 2, 2, 2, 2, 3 ),
 ( 0.1666819079834106210, 0.2000000000000000111, 0.2500000000000000000, 0.2999999999999999889, 0.3499999999999999778, 0.4000000000000000222 ),
 .UNSPECIFIED. ) 
 CURVE ( )  GEOMETRIC_REPRESENTATION_ITEM ( )  RATIONAL_B_SPLINE_CURVE ( ( 0.9945256517182514688, 0.9917959799814378696, 1.000000000000000000, 0.9876883405951377704, 1.000000000000000000, 0.9876883405951377704, 1.000000000000000000, 0.9876883405951377704, 1.000000000000000000, 0.9876883405951377704, 1.000000000000000000 ) ) 
 REPRESENTATION_ITEM ( '' )  );
#2840=ORIENTED_EDGE ( 'NONE', *, *, #9859, .F. ) ;
#2842=CARTESIAN_POINT ( 'NONE',  ( 3.143139765844590983, -4.840010801796506890, -12.50000000000000533 ) ) ;
#2848=CARTESIAN_POINT ( 'NONE',  ( 1.185096637661176677, -5.575441324182703440, -7.000000000000005329 ) ) ;
#2851=LINE ( 'NONE', #13565, #19746 ) ;
#2853=CARTESIAN_POINT ( 'NONE',  ( 3.814044456245502701, 4.235925505221138643, -11.31249999590322375 ) ) ;
#2875=LINE ( 'NONE', #5771, #17263 ) ;
#2876=CARTESIAN_POINT ( 'NONE',  ( 4.942249507334556036, -0.2590123213421313686, -9.968749997951615427 ) ) ;
#2877=CARTESIAN_POINT ( 'NONE',  ( -5.763142191869152775, 0.3020334839683282979, -10.81249999590322375 ) ) ;
#2880=DIRECTION ( 'NONE',  ( 1.000000000000000000, 0.000000000000000000, 0.000000000000000000 ) ) ;
#2893=CARTESIAN_POINT ( 'NONE',  ( -0.5958122406255597081, 5.668774803599165857, -15.31249999590322552 ) ) ;
#2910=CARTESIAN_POINT ( 'NONE',  ( -1.773574444220725077, 4.620319390059829168, -6.968749997951614539 ) ) ;
#2919=CARTESIAN_POINT ( 'NONE',  ( 3.954556930911861112, 2.873153789725825913, -14.46874999795161720 ) ) ;
#2922=CARTESIAN_POINT ( 'NONE',  ( 2.647025296875021638, 4.584782303107579615, -7.078124996927420476 ) ) ;
#2930=DIRECTION ( 'NONE',  ( 0.8090169943749512260, 0.5877852522924679191, 0.000000000000000000 ) ) ;
#2948=CARTESIAN_POINT ( 'NONE',  ( -3.814044456245531567, -4.235925505221111997, -11.31249999590322375 ) ) ;
#2950=( BOUNDED_SURFACE ( )  B_SPLINE_SURFACE ( 1, 2, ( 
 ( #15739, #9748, #634, #9848, #12833, #6408, #4932, #15838, #14035, #5026, #14335, #6709, #11036, #11340, #17439, #15938, #9542 ),
 ( #15543, #15639, #2221, #13940, #8018, #329, #1925, #232, #2027, #434, #6511, #12640, #10939, #17044, #11137, #6316, #3333 ) ),
 .UNSPECIFIED., .F., .F., .F. ) 
 B_SPLINE_SURFACE_WITH_KNOTS ( ( 2, 2 ),
 ( 3, 2, 2, 2, 2, 2, 2, 2, 3 ),
 ( 0.000000000000000000, 1.000000000000000000 ),
 ( 0.000000000000000000, 0.05000000000000000278, 0.1000000000000000056, 0.1499999999999999944, 0.2000000000000000111, 0.2500000000000000000, 0.2999999999999999889, 0.3499999999999999778, 0.4000000000000000222 ),
 .UNSPECIFIED. ) 
 GEOMETRIC_REPRESENTATION_ITEM ( )  RATIONAL_B_SPLINE_SURFACE ( (
 ( 1.000000000000000000, 0.9876883405951377704, 1.000000000000000000, 0.9876883405951377704, 1.000000000000000000, 0.9876883405951377704, 1.000000000000000000, 0.9876883405951377704, 1.000000000000000000, 0.9876883405951377704, 1.000000000000000000, 0.9876883405951377704, 1.000000000000000000, 0.9876883405951377704, 1.000000000000000000, 0.9876883405951377704, 1.000000000000000000),
 ( 1.000000000000000000, 0.9876883405951377704, 1.000000000000000000, 0.9876883405951377704, 1.000000000000000000, 0.9876883405951377704, 1.000000000000000000, 0.9876883405951377704, 1.000000000000000000, 0.9876883405951377704, 1.000000000000000000, 0.9876883405951377704, 1.000000000000000000, 0.9876883405951377704, 1.000000000000000000, 0.9876883405951377704, 1.000000000000000000) ) ) 
 REPRESENTATION_ITEM ( '' )  SURFACE ( )  );
#2969=CARTESIAN_POINT ( 'NONE',  ( -0.5109457054261112852, 4.861323657744413218, -14.84374999795161543 ) ) ;
#2981=CARTESIAN_POINT ( 'NONE',  ( 2.873153789725825025, 3.954556930911862000, -13.84374999795161543 ) ) ;
#3008=CARTESIAN_POINT ( 'NONE',  ( -4.780397808154247308, 1.280903732194486722, -13.96874999795161365 ) ) ;
#3014=CARTESIAN_POINT ( 'NONE',  ( 2.873153789725797491, -3.954556930911881985, -9.843749997951615427 ) ) ;
#3015=ORIENTED_EDGE ( 'NONE', *, *, #12236, .T. ) ;
#3017=CARTESIAN_POINT ( 'NONE',  ( -2.873153789725825469, 3.954556930911862000, -9.468749997951615427 ) ) ;
#3022=EDGE_LOOP ( 'NONE', ( #7553, #18998, #8944, #1153, #18070, #8036, #3399, #18429, #14732, #16328, #6534, #7883, #9284, #10530, #3417, #782, #10195 ) ) ;
#3044=ORIENTED_EDGE ( 'NONE', *, *, #14676, .T. ) ;
#3048=DIRECTION ( 'NONE',  ( 0.8660254037844432595, 0.4999999999999920619, -0.000000000000000000 ) ) ;
#3049=CARTESIAN_POINT ( 'NONE',  ( -5.575441324182703440, -1.185096637661177343, -13.31249999590322730 ) ) ;
#3053=CARTESIAN_POINT ( 'NONE',  ( 4.936344801571308061, 2.849999999999989875, -12.31249999590322552 ) ) ;
#3066=CARTESIAN_POINT ( 'NONE',  ( 5.699999999999994849, -0.9027913098498966393, -7.812499995903224637 ) ) ;
#3068=ORIENTED_EDGE ( 'NONE', *, *, #16920, .F. ) ;
#3079=ORIENTED_EDGE ( 'NONE', *, *, #11485, .F. ) ;
#3098=CARTESIAN_POINT ( 'NONE',  ( 0.000000000000000000, 4.200000000000000178, -28.99999999999999645 ) ) ;
#3112=ORIENTED_EDGE ( 'NONE', *, *, #3156, .T. ) ;
#3116=CARTESIAN_POINT ( 'NONE',  ( 3.499494075959792116, -3.499494075959840966, -9.343749997951615427 ) ) ;
#3122=CARTESIAN_POINT ( 'NONE',  ( 0.000000000000000000, 0.000000000000000000, -6.000000000000005329 ) ) ;
#3145=CARTESIAN_POINT ( 'NONE',  ( 4.233219804643871598, -2.444050593750019651, -11.46874999795161543 ) ) ;
#3147=CARTESIAN_POINT ( 'NONE',  ( 4.942249507334556924, 0.2590123213420971182, -12.96874999795161543 ) ) ;
#3151=CARTESIAN_POINT ( 'NONE',  ( 2.849999999999954348, -4.936344801571327601, -7.312499995903225525 ) ) ;
#3156=EDGE_CURVE ( 'NONE', #2645, #13293, #6378, .T. ) ;
#3168=ORIENTED_EDGE ( 'NONE', *, *, #14281, .T. ) ;
#3176=CARTESIAN_POINT ( 'NONE',  ( -5.700000000000000178, -2.180340287075187351E-16, -12.66727757604271076 ) ) ;
#3179=CARTESIAN_POINT ( 'NONE',  ( 0.9027913098498566713, 5.699999999999999289, -11.50000000000000355 ) ) ;
#3183=ORIENTED_EDGE ( 'NONE', *, *, #4858, .F. ) ;
#3190=ORIENTED_EDGE ( 'NONE', *, *, #18445, .T. ) ;
#3194=VERTEX_POINT ( 'NONE', #14795 ) ;
#3203=CARTESIAN_POINT ( 'NONE',  ( -4.888101187500000222, 0.7741991708318887166, -7.343749997951615427 ) ) ;
#3210=CARTESIAN_POINT ( 'NONE',  ( 3.954556930911861112, 2.873153789725825913, -14.46874999795161720 ) ) ;
#3214=CIRCLE ( 'NONE', #13439, 4.200000000000000178 ) ;
#3226=CARTESIAN_POINT ( 'NONE',  ( -4.233219804643904460, -2.444050593749961031, -11.84374999795161365 ) ) ;
#3230=PLANE ( 'NONE',  #9037 ) ;
#3253=CARTESIAN_POINT ( 'NONE',  ( 4.942249507334556924, 0.2590123213420975623, -13.34374999795161365 ) ) ;
#3260=CARTESIAN_POINT ( 'NONE',  ( 1.185096637661176677, -5.575441324182703440, -7.000000000000005329 ) ) ;
#3272=CARTESIAN_POINT ( 'NONE',  ( -5.574407415329146964, 1.493657965219562067, -14.81249999590322552 ) ) ;
#3278=CARTESIAN_POINT ( 'NONE',  ( 3.954556930911861112, 2.873153789725825913, -14.46874999795161720 ) ) ;
#3297=B_SPLINE_CURVE_WITH_KNOTS ( 'NONE', 1,
 ( #1392, #18294 ),
 .UNSPECIFIED., .F., .F.,
 ( 2, 2 ),
 ( 0.000000000000000000, 1.000000000000000000 ),
 .UNSPECIFIED. ) ;
#3310=EDGE_CURVE ( 'NONE', #6550, #4244, #760, .T. ) ;
#3326=DIRECTION ( 'NONE',  ( -0.000000000000000000, -0.000000000000000000, 1.000000000000000000 ) ) ;
#3330=CARTESIAN_POINT ( 'NONE',  ( 1.773574444220693103, -4.620319390059841602, -7.343749997951615427 ) ) ;
#3333=CARTESIAN_POINT ( 'NONE',  ( 0.5109457054261454800, -4.861323657744410554, -14.46874999795161720 ) ) ;
#3343=CARTESIAN_POINT ( 'NONE',  ( -3.846120219227966430, -3.114526743279228072, -10.96874999795161720 ) ) ;
#3364=ORIENTED_EDGE ( 'NONE', *, *, #4183, .T. ) ;
#3365=CIRCLE ( 'NONE', #15147, 9.000000000000000000 ) ;
#3381=CARTESIAN_POINT ( 'NONE',  ( -1.493657965219446382, 5.574407415329178939, -14.81249999590322552 ) ) ;
#3384=LINE ( 'NONE', #16806, #1349 ) ;
#3392=CARTESIAN_POINT ( 'NONE',  ( -5.574407415329178939, -1.493657965219446160, -9.812499995903225525 ) ) ;
#3394=CARTESIAN_POINT ( 'NONE',  ( 1.761396867937162769, -5.421022142882388373, -10.00000000000000533 ) ) ;
#3399=ORIENTED_EDGE ( 'NONE', *, *, #19726, .T. ) ;
#3402=CARTESIAN_POINT ( 'NONE',  ( 5.387740456496221242, -2.068159791354220900, -10.50000000000000533 ) ) ;
#3404=CARTESIAN_POINT ( 'NONE',  ( -2.647025296874989664, 4.584782303107598267, -6.234374998975811266 ) ) ;
#3417=ORIENTED_EDGE ( 'NONE', *, *, #2322, .T. ) ;
#3419=LINE ( 'NONE', #4721, #18086 ) ;
#3429=DIRECTION ( 'NONE',  ( -0.5877852522924721379, 0.8090169943749482284, 0.000000000000000000 ) ) ;
#3450=CARTESIAN_POINT ( 'NONE',  ( -1.493657965219562511, -5.574407415329147852, -8.500000000000007105 ) ) ;
#3454=ORIENTED_EDGE ( 'NONE', *, *, #6025, .F. ) ;
#3463=ADVANCED_FACE ( 'NONE', ( #13887 ), #14595, .T. ) ;
#3464=CARTESIAN_POINT ( 'NONE',  ( 2.068159791354145849, -5.387740456496247887, -6.500000000000005329 ) ) ;
#3470=ADVANCED_FACE ( 'NONE', ( #9441 ), #18533, .T. ) ;
#3477=CARTESIAN_POINT ( 'NONE',  ( -4.233219804643852946, 2.444050593750049405, -11.84374999795161365 ) ) ;
#3522=VECTOR ( 'NONE', #18626, 1000.000000000000000 ) ;
#3551=CARTESIAN_POINT ( 'NONE',  ( -3.846120219227901149, 3.114526743279308896, -12.34374999795161543 ) ) ;
#3569=VECTOR ( 'NONE', #12330, 1000.000000000000227 ) ;
#3570=CARTESIAN_POINT ( 'NONE',  ( -0.5109457054261112852, 4.861323657744413218, -14.84374999795161543 ) ) ;
#3580=DIRECTION ( 'NONE',  ( -0.000000000000000000, -0.000000000000000000, 1.000000000000000000 ) ) ;
#3583=CARTESIAN_POINT ( 'NONE',  ( -2.647025296875054057, -4.584782303107560963, -6.234374998975811266 ) ) ;
#3584=CARTESIAN_POINT ( 'NONE',  ( 5.699999999999994849, -0.9027913098498965283, -6.500000000000005329 ) ) ;
#3592=CARTESIAN_POINT ( 'NONE',  ( 5.387740456496233676, 2.068159791354184041, -12.81249999590322552 ) ) ;
#3593=ORIENTED_EDGE ( 'NONE', *, *, #3310, .T. ) ;
#3596=CARTESIAN_POINT ( 'NONE',  ( 3.631840208645826795, 4.484949146646356688, -7.812499995903224637 ) ) ;
#3601=( BOUNDED_CURVE ( )  B_SPLINE_CURVE ( 2, ( #17413, #11502, #13100, #6880, #8301, #6785, #19194, #3698, #992, #5298, #14801, #10016, #9918, #11694, #8407, #17604, #17800 ),
 .UNSPECIFIED., .F., .F. ) 
 B_SPLINE_CURVE_WITH_KNOTS ( ( 3, 2, 2, 2, 2, 2, 2, 2, 3 ),
 ( 0.000000000000000000, 0.05000000000000000971, 0.1000000000000000194, 0.1499999999999999944, 0.2000000000000000389, 0.2500000000000000000, 0.2999999999999999889, 0.3499999999999999223, 0.4000000000000000777 ),
 .UNSPECIFIED. ) 
 CURVE ( )  GEOMETRIC_REPRESENTATION_ITEM ( )  RATIONAL_B_SPLINE_CURVE ( ( 1.000000000000000000, 0.9876883405951377704, 1.000000000000000000, 0.9876883405951377704, 1.000000000000000000, 0.9876883405951377704, 1.000000000000000000, 0.9876883405951377704, 1.000000000000000000, 0.9876883405951377704, 1.000000000000000000, 0.9876883405951377704, 1.000000000000000000, 0.9876883405951377704, 1.000000000000000000, 0.9876883405951377704, 1.000000000000000000 ) ) 
 REPRESENTATION_ITEM ( '' )  );
#3635=CARTESIAN_POINT ( 'NONE',  ( -0.5109457054262123155, -4.861323657744403448, -8.468749997951615427 ) ) ;
#3650=CARTESIAN_POINT ( 'NONE',  ( 4.465502636338025688, -1.988169868018592412, -14.84374999795161543 ) ) ;
#3669=CARTESIAN_POINT ( 'NONE',  ( -4.620319390059805187, 1.773574444220790136, -10.96874999795161720 ) ) ;
#3683=CARTESIAN_POINT ( 'NONE',  ( 5.700000000000001954, 0.2987243419133224775, -9.165444847914525184 ) ) ;
#3689=CARTESIAN_POINT ( 'NONE',  ( 2.318398865532073749, 5.207209108562820710, -10.31249999590322552 ) ) ;
#3693=CARTESIAN_POINT ( 'NONE',  ( 4.861323657744411442, 0.5109457054261445919, -9.843749997951615427 ) ) ;
#3698=CARTESIAN_POINT ( 'NONE',  ( -2.695436003842760719, -4.150607464521772094, -10.34374999795161543 ) ) ;
#3700=EDGE_CURVE ( 'NONE', #17330, #4658, #14705, .T. ) ;
#3725=CARTESIAN_POINT ( 'NONE',  ( -5.700000000000000178, 0.9027913098498568933, -7.812499995903224637 ) ) ;
#3740=CARTESIAN_POINT ( 'NONE',  ( 4.888101187500000222, -3.413342815706642518E-14, -6.468749997951615427 ) ) ;
#3765=CARTESIAN_POINT ( 'NONE',  ( -3.114526743279308896, -3.846120219227901149, -6.968749997951614539 ) ) ;
#3770=CARTESIAN_POINT ( 'NONE',  ( -5.763142191869152775, 0.3020334839683282979, -9.500000000000003553 ) ) ;
#3777=ORIENTED_EDGE ( 'NONE', *, *, #353, .T. ) ;
#3789=ORIENTED_EDGE ( 'NONE', *, *, #10519, .T. ) ;
#3797=CARTESIAN_POINT ( 'NONE',  ( -2.246813503491833508, 4.409619785863906571, -10.34374999795161543 ) ) ;
#3818=ORIENTED_EDGE ( 'NONE', *, *, #17472, .F. ) ;
#3820=CARTESIAN_POINT ( 'NONE',  ( -4.611396867937201272, 3.350375938067097437, -9.312499995903225525 ) ) ;
#3824=CARTESIAN_POINT ( 'NONE',  ( 0.2590123213420631454, -4.942249507334558700, -8.343749997951611874 ) ) ;
#3827=VERTEX_POINT ( 'NONE', #16921 ) ;
#3831=CARTESIAN_POINT ( 'NONE',  ( 0.000000000000000000, 0.000000000000000000, 0.000000000000000000 ) ) ;
#3847=CARTESIAN_POINT ( 'NONE',  ( 1.510506337161829027, -4.648860486681964055, -10.84374999795161543 ) ) ;
#3848=CYLINDRICAL_SURFACE ( 'NONE', #10723, 5.700000000000001954 ) ;
#3853=CARTESIAN_POINT ( 'NONE',  ( -2.695436003842674122, 4.150607464521828938, -13.34374999795161365 ) ) ;
#3859=CARTESIAN_POINT ( 'NONE',  ( -1.280903732194386802, 4.780397808154273065, -13.96874999795161365 ) ) ;
#3862=LINE ( 'NONE', #8474, #10012 ) ;
#3865=CARTESIAN_POINT ( 'NONE',  ( -4.484949146646330931, 3.631840208645857437, -11.50000000000000355 ) ) ;
#3885=( BOUNDED_CURVE ( )  B_SPLINE_CURVE ( 2, ( #9257, #2112, #17323, #19020, #9157, #8216, #11221, #12922, #9631, #15724, #18819 ),
 .UNSPECIFIED., .F., .F. ) 
 B_SPLINE_CURVE_WITH_KNOTS ( ( 3, 2, 2, 2, 2, 3 ),
 ( 0.1666819079834106210, 0.2000000000000000111, 0.2500000000000000000, 0.2999999999999999889, 0.3499999999999999778, 0.4000000000000000222 ),
 .UNSPECIFIED. ) 
 CURVE ( )  GEOMETRIC_REPRESENTATION_ITEM ( )  RATIONAL_B_SPLINE_CURVE ( ( 0.9945256517182514688, 0.9917959799814378696, 1.000000000000000000, 0.9876883405951377704, 1.000000000000000000, 0.9876883405951377704, 1.000000000000000000, 0.9876883405951377704, 1.000000000000000000, 0.9876883405951377704, 1.000000000000000000 ) ) 
 REPRESENTATION_ITEM ( '' )  );
#3889=FACE_OUTER_BOUND ( 'NONE', #5653, .T. ) ;
#3894=CARTESIAN_POINT ( 'NONE',  ( 3.499494075959815653, 3.499494075959816541, -14.34374999795161543 ) ) ;
#3931=CARTESIAN_POINT ( 'NONE',  ( -3.499494075959840078, -3.499494075959791672, -14.34374999795161365 ) ) ;
#3936=EDGE_LOOP ( 'NONE', ( #18370, #13354 ) ) ;
#3945=LINE ( 'NONE', #4045, #5469 ) ;
#3947=CARTESIAN_POINT ( 'NONE',  ( 4.888101187500000222, -3.413342815706642518E-14, -6.468749997951615427 ) ) ;
#3993=CARTESIAN_POINT ( 'NONE',  ( 4.780397808154266848, 1.280903732194421218, -9.343749997951615427 ) ) ;
#4016=ADVANCED_FACE ( 'NONE', ( #17871 ), #18786, .T. ) ;
#4017=CARTESIAN_POINT ( 'NONE',  ( -5.421022142882375938, 1.761396867937200517, -8.312499995903225525 ) ) ;
#4045=CARTESIAN_POINT ( 'NONE',  ( -5.207209108562805611, 2.318398865532109276, 0.000000000000000000 ) ) ;
#4058=ORIENTED_EDGE ( 'NONE', *, *, #19726, .F. ) ;
#4059=CARTESIAN_POINT ( 'NONE',  ( -0.5109457054261112852, 4.861323657744413218, -14.46874999795161720 ) ) ;
#4063=ORIENTED_EDGE ( 'NONE', *, *, #9147, .F. ) ;
#4092=CARTESIAN_POINT ( 'NONE',  ( -5.575441324182679459, 1.185096637661293251, -10.00000000000000533 ) ) ;
#4094=CARTESIAN_POINT ( 'NONE',  ( 1.280903732194421440, -4.780397808154265071, -13.96874999795161365 ) ) ;
#4096=ORIENTED_EDGE ( 'NONE', *, *, #6801, .T. ) ;
#4106=DIRECTION ( 'NONE',  ( 1.000000000000000000, 0.000000000000000000, 0.000000000000000000 ) ) ;
#4117=CARTESIAN_POINT ( 'NONE',  ( -0.9027913098498572264, 5.700000000000000178, -10.50000000000000533 ) ) ;
#4119=CARTESIAN_POINT ( 'NONE',  ( 2.444050593749960587, -4.233219804643904460, -6.468749997951615427 ) ) ;
#4120=CARTESIAN_POINT ( 'NONE',  ( 5.700000000000001066, -3.980288726281172656E-14, -6.656249997951614539 ) ) ;
#4123=( BOUNDED_CURVE ( )  B_SPLINE_CURVE ( 2, ( #18534, #12438, #17139, #10837, #13839, #15638, #1536, #9443, #9241 ),
 .UNSPECIFIED., .F., .F. ) 
 B_SPLINE_CURVE_WITH_KNOTS ( ( 3, 2, 2, 2, 3 ),
 ( 0.000000000000000000, 0.05000000000000000278, 0.1000000000000000056, 0.1499999999999999944, 0.1666819079834106210 ),
 .UNSPECIFIED. ) 
 CURVE ( )  GEOMETRIC_REPRESENTATION_ITEM ( )  RATIONAL_B_SPLINE_CURVE ( ( 1.000000000000000000, 0.9876883405951377704, 1.000000000000000000, 0.9876883405951377704, 1.000000000000000000, 0.9876883405951377704, 1.000000000000000000, 0.9958923606136999007, 0.9945256517182514688 ) ) 
 REPRESENTATION_ITEM ( '' )  );
#4126=CARTESIAN_POINT ( 'NONE',  ( 0.9027913098498173694, -5.700000000000005507, -11.81249999590322552 ) ) ;
#4130=FACE_OUTER_BOUND ( 'NONE', #652, .T. ) ;
#4156=CARTESIAN_POINT ( 'NONE',  ( -4.861323657744413218, -0.5109457054261099529, -9.843749997951615427 ) ) ;
#4158=CARTESIAN_POINT ( 'NONE',  ( 2.318398865532074193, 5.207209108562820710, -9.000000000000005329 ) ) ;
#4183=EDGE_CURVE ( 'NONE', #768, #3194, #9515, .T. ) ;
#4204=CARTESIAN_POINT ( 'NONE',  ( 4.781284448697187273, -1.016293382781444654, -10.84374999795161543 ) ) ;
#4217=CARTESIAN_POINT ( 'NONE',  ( -1.988169868018624609, -4.465502636338009701, -9.843749997951615427 ) ) ;
#4218=DIRECTION ( 'NONE',  ( 0.000000000000000000, 0.000000000000000000, -1.000000000000000000 ) ) ;
#4220=VERTEX_POINT ( 'NONE', #16063 ) ;
#4238=( NAMED_UNIT ( * ) PLANE_ANGLE_UNIT ( ) SI_UNIT ( $, .RADIAN. ) );
#4244=VERTEX_POINT ( 'NONE', #1146 ) ;
#4246=( BOUNDED_CURVE ( )  B_SPLINE_CURVE ( 2, ( #14163, #9673, #5253, #8047, #12863, #18661, #2053, #14266, #17265, #2154, #8259, #3551, #354, #3853, #11369, #15771, #15667 ),
 .UNSPECIFIED., .F., .F. ) 
 B_SPLINE_CURVE_WITH_KNOTS ( ( 3, 2, 2, 2, 2, 2, 2, 2, 3 ),
 ( 0.000000000000000000, 0.05000000000000000971, 0.1000000000000000194, 0.1499999999999999944, 0.2000000000000000389, 0.2500000000000000000, 0.2999999999999999889, 0.3499999999999999223, 0.4000000000000000777 ),
 .UNSPECIFIED. ) 
 CURVE ( )  GEOMETRIC_REPRESENTATION_ITEM ( )  RATIONAL_B_SPLINE_CURVE ( ( 1.000000000000000000, 0.9876883405951377704, 1.000000000000000000, 0.9876883405951377704, 1.000000000000000000, 0.9876883405951377704, 1.000000000000000000, 0.9876883405951377704, 1.000000000000000000, 0.9876883405951377704, 1.000000000000000000, 0.9876883405951377704, 1.000000000000000000, 0.9876883405951377704, 1.000000000000000000, 0.9876883405951377704, 1.000000000000000000 ) ) 
 REPRESENTATION_ITEM ( '' )  );
#4253=CARTESIAN_POINT ( 'NONE',  ( 4.780397808154266848, 1.280903732194421218, -8.968749997951611874 ) ) ;
#4260=CARTESIAN_POINT ( 'NONE',  ( -3.846120219227966430, -3.114526743279228072, -10.96874999795161720 ) ) ;
#4276=CARTESIAN_POINT ( 'NONE',  ( 4.465502636338025688, -1.988169868018592856, -14.46874999795161720 ) ) ;
#4287=CARTESIAN_POINT ( 'NONE',  ( -3.143139765844555900, 4.840010801796527318, -12.50000000000000533 ) ) ;
#4294=ORIENTED_EDGE ( 'NONE', *, *, #10908, .F. ) ;
#4316=CARTESIAN_POINT ( 'NONE',  ( -2.695436003842760275, -4.150607464521772094, -10.34374999795161543 ) ) ;
#4322=CARTESIAN_POINT ( 'NONE',  ( -2.246813503491864150, -4.409619785863891472, -13.34374999795161365 ) ) ;
#4326=CARTESIAN_POINT ( 'NONE',  ( 0.5109457054261784537, 4.861323657744407001, -8.468749997951615427 ) ) ;
#4336=SURFACE_SIDE_STYLE ('',( #16546 ) ) ;
#4339=CARTESIAN_POINT ( 'NONE',  ( 2.873153789725797491, -3.954556930911881985, -9.468749997951615427 ) ) ;
#4355=ORIENTED_EDGE ( 'NONE', *, *, #163, .F. ) ;
#4356=CARTESIAN_POINT ( 'NONE',  ( -1.016293382781411125, 4.781284448697194378, -7.468749997951615427 ) ) ;
#4359=CARTESIAN_POINT ( 'NONE',  ( 2.849999999999954348, -4.936344801571327601, -6.000000000000005329 ) ) ;
#4362=VERTEX_POINT ( 'NONE', #16552 ) ;
#4377=CARTESIAN_POINT ( 'NONE',  ( -4.080749450109677490, -4.080749450109622423, -14.81249999590322375 ) ) ;
#4387=CARTESIAN_POINT ( 'NONE',  ( -5.575441324182679459, 1.185096637661293251, -11.31249999590322375 ) ) ;
#4391=CARTESIAN_POINT ( 'NONE',  ( -3.114526743279308896, -3.846120219227900705, -6.968749997951614539 ) ) ;
#4422=CARTESIAN_POINT ( 'NONE',  ( 4.781284448697194378, 1.016293382781411792, -12.84374999795161543 ) ) ;
#4449=CARTESIAN_POINT ( 'NONE',  ( 1.280903732194421663, -4.780397808154265960, -13.96874999795161365 ) ) ;
#4456=CARTESIAN_POINT ( 'NONE',  ( 5.575441324182695446, 1.185096637661215757, -12.00000000000000533 ) ) ;
#4461=DIRECTION ( 'NONE',  ( -0.000000000000000000, -0.000000000000000000, 1.000000000000000000 ) ) ;
#4469=CARTESIAN_POINT ( 'NONE',  ( 2.444050593749960587, -4.233219804643904460, -6.843749997951615427 ) ) ;
#4472=ORIENTED_EDGE ( 'NONE', *, *, #16768, .F. ) ;
#4490=ADVANCED_FACE ( 'NONE', ( #9642 ), #2950, .T. ) ;
#4503=EDGE_CURVE ( 'NONE', #13431, #12853, #1670, .T. ) ;
#4511=CARTESIAN_POINT ( 'NONE',  ( -4.888101187500000222, 0.000000000000000000, -6.468749997951615427 ) ) ;
#4512=CARTESIAN_POINT ( 'NONE',  ( 4.409619785863891472, -2.246813503491864150, -8.343749997951613651 ) ) ;
#4514=CARTESIAN_POINT ( 'NONE',  ( 2.695436003842732298, 4.150607464521791634, -9.968749997951617203 ) ) ;
#4539=FACE_OUTER_BOUND ( 'NONE', #17616, .T. ) ;
#4540=LINE ( 'NONE', #15053, #7761 ) ;
#4541=ORIENTED_EDGE ( 'NONE', *, *, #6214, .T. ) ;
#4545=CARTESIAN_POINT ( 'NONE',  ( 5.387740456496221242, -2.068159791354221344, -10.50000000000000711 ) ) ;
#4552=CARTESIAN_POINT ( 'NONE',  ( -5.387740456496247887, -2.068159791354146293, -12.81249999590322552 ) ) ;
#4576=LINE ( 'NONE', #12180, #11421 ) ;
#4579=VERTEX_POINT ( 'NONE', #11622 ) ;
#4592=CARTESIAN_POINT ( 'NONE',  ( -5.700000000000001066, 0.2987243419133610023, -14.14705514798868435 ) ) ;
#4611=ORIENTED_EDGE ( 'NONE', *, *, #13125, .T. ) ;
#4618=CARTESIAN_POINT ( 'NONE',  ( -2.873153789725825469, 3.954556930911862000, -9.843749997951615427 ) ) ;
#4620=ORIENTED_EDGE ( 'NONE', *, *, #13728, .T. ) ;
#4643=ORIENTED_EDGE ( 'NONE', *, *, #12019, .F. ) ;
#4646=CARTESIAN_POINT ( 'NONE',  ( 0.5958122406255995651, -5.668774803599162304, -14.00000000000000533 ) ) ;
#4649=EDGE_CURVE ( 'NONE', #14057, #11278, #2190, .T. ) ;
#4653=CARTESIAN_POINT ( 'NONE',  ( 3.846120219227944670, 3.114526743279255161, -10.96874999795161720 ) ) ;
#4655=PRODUCT_CONTEXT ( 'NONE', #15199, 'mechanical' ) ;
#4658=VERTEX_POINT ( 'NONE', #8818 ) ;
#4660=CARTESIAN_POINT ( 'NONE',  ( -0.2590123213420975623, 4.942249507334556924, -8.343749997951611874 ) ) ;
#4661=VERTEX_POINT ( 'NONE', #13412 ) ;
#4668=DIRECTION ( 'NONE',  ( 0.000000000000000000, -1.000000000000000000, 0.000000000000000000 ) ) ;
#4670=CARTESIAN_POINT ( 'NONE',  ( -4.611396867937224364, -3.350375938067065906, -15.31249999590322552 ) ) ;
#4684=CARTESIAN_POINT ( 'NONE',  ( -3.846120219227901593, 3.114526743279308896, -12.34374999795161543 ) ) ;
#4716=AXIS2_PLACEMENT_3D ( 'NONE', #3098, #15608, #1894 ) ;
#4721=CARTESIAN_POINT ( 'NONE',  ( 4.888101187500000222, -3.413342815706642518E-14, -6.656249997951614539 ) ) ;
#4726=CARTESIAN_POINT ( 'NONE',  ( 2.318398865532038666, -5.207209108562836697, -14.31249999590322552 ) ) ;
#4729=CARTESIAN_POINT ( 'NONE',  ( -1.280903732194487166, -4.780397808154247308, -9.343749997951615427 ) ) ;
#4754=CARTESIAN_POINT ( 'NONE',  ( 1.280903732194454081, 4.780397808154257078, -9.343749997951615427 ) ) ;
#4761=( BOUNDED_CURVE ( )  B_SPLINE_CURVE ( 2, ( #3740, #5617, #15851, #8242, #17550, #14348, #11635, #647, #6721, #19045, #12950, #9957, #2235, #5335, #16048, #11539, #17644 ),
 .UNSPECIFIED., .F., .F. ) 
 B_SPLINE_CURVE_WITH_KNOTS ( ( 3, 2, 2, 2, 2, 2, 2, 2, 3 ),
 ( 0.000000000000000000, 0.05000000000000000971, 0.1000000000000000194, 0.1499999999999999944, 0.2000000000000000389, 0.2500000000000000000, 0.2999999999999999889, 0.3499999999999999223, 0.4000000000000000777 ),
 .UNSPECIFIED. ) 
 CURVE ( )  GEOMETRIC_REPRESENTATION_ITEM ( )  RATIONAL_B_SPLINE_CURVE ( ( 1.000000000000000000, 0.9876883405951377704, 1.000000000000000000, 0.9876883405951377704, 1.000000000000000000, 0.9876883405951377704, 1.000000000000000000, 0.9876883405951377704, 1.000000000000000000, 0.9876883405951377704, 1.000000000000000000, 0.9876883405951377704, 1.000000000000000000, 0.9876883405951377704, 1.000000000000000000, 0.9876883405951377704, 1.000000000000000000 ) ) 
 REPRESENTATION_ITEM ( '' )  );
#4769=VERTEX_POINT ( 'NONE', #17018 ) ;
#4773=EDGE_LOOP ( 'NONE', ( #18932, #11027, #13859, #7229 ) ) ;
#4781=CARTESIAN_POINT ( 'NONE',  ( -4.861323657744413218, -0.5109457054261099529, -9.843749997951615427 ) ) ;
#4831=DIRECTION ( 'NONE',  ( 0.4067366430758020401, 0.9135454576426000894, 0.000000000000000000 ) ) ;
#4838=CARTESIAN_POINT ( 'NONE',  ( -1.280903732194487166, -4.780397808154247308, -8.968749997951613651 ) ) ;
#4849=CARTESIAN_POINT ( 'NONE',  ( -0.5958122406256771697, -5.668774803599153422, -8.000000000000005329 ) ) ;
#4855=LINE ( 'NONE', #7754, #924 ) ;
#4856=CARTESIAN_POINT ( 'NONE',  ( 5.668774803599156975, -0.5958122406256373127, -14.31249999590322552 ) ) ;
#4858=EDGE_CURVE ( 'NONE', #12027, #5756, #11022, .T. ) ;
#4874=CARTESIAN_POINT ( 'NONE',  ( 4.611396867937200383, 3.350375938067097881, -14.00000000000000533 ) ) ;
#4876=CARTESIAN_POINT ( 'NONE',  ( -1.493657965219562511, -5.574407415329147852, -9.812499995903223748 ) ) ;
#4877=CARTESIAN_POINT ( 'NONE',  ( -5.207209108562804722, 2.318398865532109276, -14.00000000000000533 ) ) ;
#4881=CARTESIAN_POINT ( 'NONE',  ( -4.150607464521828938, -2.695436003842674566, -8.343749997951611874 ) ) ;
#4885=( BOUNDED_CURVE ( )  B_SPLINE_CURVE ( 2, ( #3176, #13985, #275, #6357, #4877 ),
 .UNSPECIFIED., .F., .F. ) 
 B_SPLINE_CURVE_WITH_KNOTS ( ( 3, 2, 3 ),
 ( 0.3333180920165860761, 0.3499999999999999778, 0.4000000000000000222 ),
 .UNSPECIFIED. ) 
 CURVE ( )  GEOMETRIC_REPRESENTATION_ITEM ( )  RATIONAL_B_SPLINE_CURVE ( ( 0.9945256517182510247, 0.9958923606136991236, 1.000000000000000000, 0.9876883405951377704, 1.000000000000000000 ) ) 
 REPRESENTATION_ITEM ( '' )  );
#4890=EDGE_CURVE ( 'NONE', #19252, #4244, #3601, .T. ) ;
#4892=CARTESIAN_POINT ( 'NONE',  ( -4.840010801796527318, -3.143139765844555900, -8.812499995903225525 ) ) ;
#4894=CARTESIAN_POINT ( 'NONE',  ( 4.888101187499994893, -0.7741991708319229115, -6.968749997951614539 ) ) ;
#4898=CARTESIAN_POINT ( 'NONE',  ( 0.000000000000000000, 0.000000000000000000, 0.000000000000000000 ) ) ;
#4911=DIRECTION ( 'NONE',  ( -0.000000000000000000, -0.000000000000000000, 1.000000000000000000 ) ) ;
#4922=ADVANCED_FACE ( 'NONE', ( #5483 ), #11144, .T. ) ;
#4932=CARTESIAN_POINT ( 'NONE',  ( 4.861323657744411442, 0.5109457054261445919, -9.843749997951615427 ) ) ;
#4961=CARTESIAN_POINT ( 'NONE',  ( 0.5109457054261454800, -4.861323657744410554, -14.84374999795161543 ) ) ;
#4977=CARTESIAN_POINT ( 'NONE',  ( -4.484949146646330931, 3.631840208645857437, -12.81249999590322552 ) ) ;
#4981=DIRECTION ( 'NONE',  ( 1.000000000000000000, 0.000000000000000000, 0.000000000000000000 ) ) ;
#4988=CARTESIAN_POINT ( 'NONE',  ( 4.611396867937178179, -3.350375938067129855, -8.000000000000005329 ) ) ;
#4997=CARTESIAN_POINT ( 'NONE',  ( 0.5958122406255995651, -5.668774803599162304, -14.00000000000000533 ) ) ;
#4999=LINE ( 'NONE', #2922, #10832 ) ;
#5002=ORIENTED_EDGE ( 'NONE', *, *, #15249, .T. ) ;
#5020=CARTESIAN_POINT ( 'NONE',  ( 3.814044456245474279, -4.235925505221167064, -13.31249999590322730 ) ) ;
#5023=CARTESIAN_POINT ( 'NONE',  ( -4.620319390059841602, -1.773574444220693325, -12.34374999795161543 ) ) ;
#5026=CARTESIAN_POINT ( 'NONE',  ( 4.620319390059819398, -1.773574444220757274, -11.34374999795161543 ) ) ;
#5030=ADVANCED_FACE ( 'NONE', ( #13389 ), #17915, .T. ) ;
#5032=ORIENTED_EDGE ( 'NONE', *, *, #13746, .T. ) ;
#5041=ADVANCED_FACE ( 'NONE', ( #8176 ), #15115, .T. ) ;
#5046=CARTESIAN_POINT ( 'NONE',  ( -4.484949146646406426, -3.631840208645764179, -10.50000000000000711 ) ) ;
#5067=CARTESIAN_POINT ( 'NONE',  ( -0.5109457054261112852, 4.861323657744413218, -14.46874999795161720 ) ) ;
#5070=CARTESIAN_POINT ( 'NONE',  ( -5.700000000000001066, 0.000000000000000000, -6.000000000000005329 ) ) ;
#5082=CARTESIAN_POINT ( 'NONE',  ( 5.700000000000002842, 2.725425358843983450E-16, -9.332722423957255486 ) ) ;
#5092=CARTESIAN_POINT ( 'NONE',  ( 0.5958122406255995651, -5.668774803599162304, -14.00000000000000533 ) ) ;
#5093=ORIENTED_EDGE ( 'NONE', *, *, #17146, .T. ) ;
#5128=CARTESIAN_POINT ( 'NONE',  ( -4.620319390059842490, -1.773574444220693325, -11.96874999795161365 ) ) ;
#5133=EDGE_LOOP ( 'NONE', ( #8441, #9065, #2718, #15843 ) ) ;
#5136=ORIENTED_EDGE ( 'NONE', *, *, #10236, .F. ) ;
#5150=CARTESIAN_POINT ( 'NONE',  ( -5.575441324182703440, -1.185096637661177343, -12.00000000000000533 ) ) ;
#5158=CARTESIAN_POINT ( 'NONE',  ( 3.270778111535338262, 3.632567103900523620, -10.46874999795161720 ) ) ;
#5163=CARTESIAN_POINT ( 'NONE',  ( 2.444050593750020095, 4.233219804643871598, -6.843749997951615427 ) ) ;
#5182=SURFACE_STYLE_USAGE ( .BOTH. , #500 ) ;
#5183=CYLINDRICAL_SURFACE ( 'NONE', #7071, 5.700000000000001954 ) ;
#5202=LINE ( 'NONE', #9826, #9428 ) ;
#5204=EDGE_CURVE ( 'NONE', #1899, #2597, #32, .T. ) ;
#5220=CARTESIAN_POINT ( 'NONE',  ( -3.490243377569957047E-16, 5.700000000000001066, -12.31249999590322552 ) ) ;
#5233=CARTESIAN_POINT ( 'NONE',  ( -3.270778111535363131, -3.632567103900500971, -10.46874999795161720 ) ) ;
#5235=CARTESIAN_POINT ( 'NONE',  ( -4.611396867937224364, -3.350375938067065906, -14.00000000000000533 ) ) ;
#5242=VERTEX_POINT ( 'NONE', #5658 ) ;
#5247=CARTESIAN_POINT ( 'NONE',  ( 3.499494075959791672, -3.499494075959840966, -9.343749997951615427 ) ) ;
#5253=CARTESIAN_POINT ( 'NONE',  ( -3.632567103900569361, -3.270778111535287191, -7.843749997951614539 ) ) ;
#5267=VERTEX_POINT ( 'NONE', #16374 ) ;
#5284=CARTESIAN_POINT ( 'NONE',  ( 5.421022142882364392, -1.761396867937238486, -7.000000000000005329 ) ) ;
#5290=CARTESIAN_POINT ( 'NONE',  ( -2.068159791354183596, 5.387740456496234565, -7.812499995903224637 ) ) ;
#5295=CARTESIAN_POINT ( 'NONE',  ( 2.850000000000024070, 4.936344801571289409, -7.312499995903225525 ) ) ;
#5297=DIRECTION ( 'NONE',  ( -0.9945218953682746221, -0.1045284632676418413, 0.000000000000000000 ) ) ;
#5298=CARTESIAN_POINT ( 'NONE',  ( -3.846120219227966430, -3.114526743279228072, -11.34374999795161543 ) ) ;
#5300=ADVANCED_FACE ( 'NONE', ( #13366 ), #5954, .T. ) ;
#5303=CARTESIAN_POINT ( 'NONE',  ( 5.574407415329170057, 1.493657965219485018, -9.812499995903225525 ) ) ;
#5309=CARTESIAN_POINT ( 'NONE',  ( -3.954556930911881096, -2.873153789725797935, -14.84374999795161543 ) ) ;
#5312=CARTESIAN_POINT ( 'NONE',  ( 4.150607464521811174, 2.695436003842704764, -8.343749997951613651 ) ) ;
#5323=CARTESIAN_POINT ( 'NONE',  ( -5.421022142882375938, 1.761396867937200517, -7.000000000000005329 ) ) ;
#5332=CARTESIAN_POINT ( 'NONE',  ( -3.350375938067128967, -4.611396867937178179, -14.31249999590322552 ) ) ;
#5335=CARTESIAN_POINT ( 'NONE',  ( -2.246813503491864150, -4.409619785863891472, -12.96874999795161543 ) ) ;
#5343=ORIENTED_EDGE ( 'NONE', *, *, #17045, .T. ) ;
#5344=CARTESIAN_POINT ( 'NONE',  ( 2.873153789725797491, -3.954556930911881985, -9.843749997951615427 ) ) ;
#5353=AXIS2_PLACEMENT_3D ( 'NONE', #15730, #3326, #12339 ) ;
#5359=CARTESIAN_POINT ( 'NONE',  ( -1.280903732194386802, 4.780397808154273065, -14.34374999795161365 ) ) ;
#5361=CARTESIAN_POINT ( 'NONE',  ( -1.016293382781411125, 4.781284448697194378, -7.468749997951615427 ) ) ;
#5364=CARTESIAN_POINT ( 'NONE',  ( -3.632567103900569361, -3.270778111535287191, -7.468749997951615427 ) ) ;
#5395=VERTEX_POINT ( 'NONE', #14440 ) ;
#5399=VERTEX_POINT ( 'NONE', #2031 ) ;
#5402=CARTESIAN_POINT ( 'NONE',  ( 0.000000000000000000, 0.000000000000000000, 0.000000000000000000 ) ) ;
#5409=LINE ( 'NONE', #14533, #1609 ) ;
#5424=CARTESIAN_POINT ( 'NONE',  ( 0.7741991708318548548, -4.888101187500005551, -11.34374999795161543 ) ) ;
#5426=EDGE_LOOP ( 'NONE', ( #2013, #10250, #10231, #13046 ) ) ;
#5429=CARTESIAN_POINT ( 'NONE',  ( -0.9027913098498963063, -5.699999999999994849, -11.50000000000000355 ) ) ;
#5449=EDGE_LOOP ( 'NONE', ( #13982, #3168, #10333, #2840 ) ) ;
#5455=CARTESIAN_POINT ( 'NONE',  ( -3.846120219227901593, 3.114526743279308896, -12.34374999795161543 ) ) ;
#5458=CARTESIAN_POINT ( 'NONE',  ( -2.695436003842674566, 4.150607464521828938, -12.96874999795161543 ) ) ;
#5461=CARTESIAN_POINT ( 'NONE',  ( 1.493657965219523875, 5.574407415329157622, -8.500000000000005329 ) ) ;
#5469=VECTOR ( 'NONE', #11839, 1000.000000000000000 ) ;
#5479=CARTESIAN_POINT ( 'NONE',  ( -4.465502636338010589, 1.988169868018623720, -14.84374999795161543 ) ) ;
#5483=FACE_OUTER_BOUND ( 'NONE', #7418, .T. ) ;
#5493=CARTESIAN_POINT ( 'NONE',  ( -5.700000000000001066, 0.000000000000000000, -7.312499995903225525 ) ) ;
#5497=AXIS2_PLACEMENT_3D ( 'NONE', #8300, #5297, #19006 ) ;
#5519=( BOUNDED_CURVE ( )  B_SPLINE_CURVE ( 2, ( #18505, #7795, #11101, #12505, #16823 ),
 .UNSPECIFIED., .F., .F. ) 
 B_SPLINE_CURVE_WITH_KNOTS ( ( 3, 2, 3 ),
 ( 0.3333180920165871863, 0.3499999999999999778, 0.4000000000000000222 ),
 .UNSPECIFIED. ) 
 CURVE ( )  GEOMETRIC_REPRESENTATION_ITEM ( )  RATIONAL_B_SPLINE_CURVE ( ( 0.9945256517182510247, 0.9958923606136993456, 1.000000000000000000, 0.9876883405951377704, 1.000000000000000000 ) ) 
 REPRESENTATION_ITEM ( '' )  );
#5524=VERTEX_POINT ( 'NONE', #8531 ) ;
#5527=CARTESIAN_POINT ( 'NONE',  ( -3.945386292505473391E-14, -5.700000000000001066, -11.00000000000000711 ) ) ;
#5542=EDGE_CURVE ( 'NONE', #488, #736, #8622, .T. ) ;
#5563=CARTESIAN_POINT ( 'NONE',  ( 0.5109457054261454800, -4.861323657744410554, -14.84374999795161543 ) ) ;
#5609=CARTESIAN_POINT ( 'NONE',  ( -2.695436003842760275, -4.150607464521772094, -9.968749997951617203 ) ) ;
#5616=CARTESIAN_POINT ( 'NONE',  ( 4.235925505221166176, 3.814044456245473835, -7.000000000000005329 ) ) ;
#5617=CARTESIAN_POINT ( 'NONE',  ( 4.888101187499994893, -0.7741991708319229115, -6.968749997951614539 ) ) ;
#5630=CARTESIAN_POINT ( 'NONE',  ( -1.510506337161893642, -4.648860486681943627, -12.46874999795161543 ) ) ;
#5650=CARTESIAN_POINT ( 'NONE',  ( 5.387740456496232788, 2.068159791354184041, -11.50000000000000355 ) ) ;
#5653=EDGE_LOOP ( 'NONE', ( #4620, #5850, #1556, #11471, #3454 ) ) ;
#5658=CARTESIAN_POINT ( 'NONE',  ( -4.888101187500000222, 0.000000000000000000, -6.468749997951615427 ) ) ;
#5662=CIRCLE ( 'NONE', #5353, 5.700000000000001954 ) ;
#5700=CARTESIAN_POINT ( 'NONE',  ( -3.954556930911881096, -2.873153789725797935, -14.84374999795161543 ) ) ;
#5709=CARTESIAN_POINT ( 'NONE',  ( -1.761396867937238042, -5.421022142882365280, -13.31249999590322730 ) ) ;
#5713=CARTESIAN_POINT ( 'NONE',  ( 1.280903732194454303, 4.780397808154257078, -9.343749997951615427 ) ) ;
#5714=LINE ( 'NONE', #14934, #12979 ) ;
#5717=EDGE_LOOP ( 'NONE', ( #14080, #17671, #6970, #2222 ) ) ;
#5723=FILL_AREA_STYLE_COLOUR ( '', #14708 ) ;
#5743=CARTESIAN_POINT ( 'NONE',  ( -2.849999999999988987, 4.936344801571308061, -6.000000000000005329 ) ) ;
#5752=CARTESIAN_POINT ( 'NONE',  ( 5.700000000000001066, 0.5990941410143489909, -12.33180101230371584 ) ) ;
#5754=CARTESIAN_POINT ( 'NONE',  ( -2.850000000000058265, -4.936344801571268093, -7.312499995903225525 ) ) ;
#5756=VERTEX_POINT ( 'NONE', #214 ) ;
#5761=CARTESIAN_POINT ( 'NONE',  ( -4.465502636338010589, 1.988169868018623720, -14.84374999795161543 ) ) ;
#5771=CARTESIAN_POINT ( 'NONE',  ( 4.611396867937201272, 3.350375938067098325, 0.000000000000000000 ) ) ;
#5799=B_SPLINE_CURVE_WITH_KNOTS ( 'NONE', 1,
 ( #8353, #3650 ),
 .UNSPECIFIED., .F., .F.,
 ( 2, 2 ),
 ( 0.000000000000000000, 1.000000000000000000 ),
 .UNSPECIFIED. ) ;
#5810=DIRECTION ( 'NONE',  ( 0.000000000000000000, 0.000000000000000000, -1.000000000000000000 ) ) ;
#5812=CARTESIAN_POINT ( 'NONE',  ( 4.861323657744406113, -0.5109457054261780096, -13.84374999795161543 ) ) ;
#5824=LINE ( 'NONE', #10642, #13454 ) ;
#5826=CARTESIAN_POINT ( 'NONE',  ( -2.873153789725852558, -3.954556930911842016, -13.84374999795161543 ) ) ;
#5841=CARTESIAN_POINT ( 'NONE',  ( 4.781284448697187273, -1.016293382781444654, -10.46874999795161720 ) ) ;
#5846=CARTESIAN_POINT ( 'NONE',  ( -4.233219804643904460, -2.444050593749961031, -11.46874999795161543 ) ) ;
#5850=ORIENTED_EDGE ( 'NONE', *, *, #1908, .T. ) ;
#5855=CARTESIAN_POINT ( 'NONE',  ( -5.021782490506605967, 2.235841616153737998, -14.11718749948790830 ) ) ;
#5861=VERTEX_POINT ( 'NONE', #12716 ) ;
#5873=ADVANCED_FACE ( 'NONE', ( #1810 ), #15817, .T. ) ;
#5892=AXIS2_PLACEMENT_3D ( 'NONE', #6028, #7830, #2930 ) ;
#5899=ORIENTED_EDGE ( 'NONE', *, *, #18807, .F. ) ;
#5904=CARTESIAN_POINT ( 'NONE',  ( 3.270778111535338262, 3.632567103900524064, -10.84374999795161543 ) ) ;
#5906=CARTESIAN_POINT ( 'NONE',  ( -4.942249507334558700, -0.2590123213420631454, -12.96874999795161543 ) ) ;
#5911=CARTESIAN_POINT ( 'NONE',  ( -4.648860486681953397, 1.510506337161861445, -7.843749997951614539 ) ) ;
#5938=DIRECTION ( 'NONE',  ( 0.8660254037844398178, 0.000000000000000000, 0.4999999999999979461 ) ) ;
#5954=PLANE ( 'NONE',  #19349 ) ;
#5977=CARTESIAN_POINT ( 'NONE',  ( -1.988169868018530906, 4.465502636338051445, -13.46874999795161543 ) ) ;
#5986=VERTEX_POINT ( 'NONE', #903 ) ;
#6000=CARTESIAN_POINT ( 'NONE',  ( -4.861323657744403448, 0.5109457054262118714, -13.84374999795161543 ) ) ;
#6007=CARTESIAN_POINT ( 'NONE',  ( -4.409619785863906571, 2.246813503491833508, -8.343749997951611874 ) ) ;
#6008=CARTESIAN_POINT ( 'NONE',  ( 4.648860486681943627, -1.510506337161893864, -7.843749997951614539 ) ) ;
#6009=ORIENTED_EDGE ( 'NONE', *, *, #14676, .F. ) ;
#6010=CARTESIAN_POINT ( 'NONE',  ( 4.780397808154257078, -1.280903732194453859, -14.34374999795161365 ) ) ;
#6025=EDGE_CURVE ( 'NONE', #4362, #1514, #15874, .T. ) ;
#6028=CARTESIAN_POINT ( 'NONE',  ( -4.447186883680888769, -3.231070400981749025, -14.11718749948790830 ) ) ;
#6040=SHAPE_REPRESENTATION ( 'DRIVER', ( #16724 ), #15776 ) ;
#6043=CARTESIAN_POINT ( 'NONE',  ( 4.936344801571308061, 2.849999999999989431, -11.00000000000000711 ) ) ;
#6049=ORIENTED_EDGE ( 'NONE', *, *, #10527, .F. ) ;
#6052=CARTESIAN_POINT ( 'NONE',  ( 5.700000000000001066, -4.360680574150373717E-16, -12.66727757604273386 ) ) ;
#6073=CARTESIAN_POINT ( 'NONE',  ( -1.510506337161861667, 4.648860486681953397, -10.84374999795161543 ) ) ;
#6078=EDGE_LOOP ( 'NONE', ( #15791, #1821, #5343, #13029, #14151 ) ) ;
#6088=DIRECTION ( 'NONE',  ( -0.000000000000000000, -0.000000000000000000, 1.000000000000000000 ) ) ;
#6098=CARTESIAN_POINT ( 'NONE',  ( 1.988169868018593300, 4.465502636338024800, -9.843749997951615427 ) ) ;
#6104=ADVANCED_FACE ( 'NONE', ( #9199 ), #12195, .T. ) ;
#6113=CARTESIAN_POINT ( 'NONE',  ( -1.510506337161861667, 4.648860486681953397, -10.46874999795161720 ) ) ;
#6137=CARTESIAN_POINT ( 'NONE',  ( 3.846120219227923798, -3.114526743279282250, -11.96874999795161365 ) ) ;
#6143=CARTESIAN_POINT ( 'NONE',  ( -5.207209108562804722, 2.318398865532109276, -14.00000000000000533 ) ) ;
#6155=ORIENTED_EDGE ( 'NONE', *, *, #4649, .T. ) ;
#6158=( BOUNDED_SURFACE ( )  B_SPLINE_SURFACE ( 1, 2, ( 
 ( #19258, #958, #7036, #16269, #17473, #17672, #4156, #8369, #11472, #10078, #1059, #5455, #13167, #16177, #14482, #5359, #8760 ),
 ( #14577, #3765, #14864, #9885, #19065, #772, #11661, #2447, #18968, #6745, #8472, #13265, #17573, #11565, #19355, #3859, #4059 ) ),
 .UNSPECIFIED., .F., .F., .F. ) 
 B_SPLINE_SURFACE_WITH_KNOTS ( ( 2, 2 ),
 ( 3, 2, 2, 2, 2, 2, 2, 2, 3 ),
 ( 0.000000000000000000, 1.000000000000000000 ),
 ( 0.000000000000000000, 0.05000000000000000278, 0.1000000000000000056, 0.1499999999999999944, 0.2000000000000000111, 0.2500000000000000000, 0.2999999999999999889, 0.3499999999999999778, 0.4000000000000000222 ),
 .UNSPECIFIED. ) 
 GEOMETRIC_REPRESENTATION_ITEM ( )  RATIONAL_B_SPLINE_SURFACE ( (
 ( 1.000000000000000000, 0.9876883405951377704, 1.000000000000000000, 0.9876883405951377704, 1.000000000000000000, 0.9876883405951377704, 1.000000000000000000, 0.9876883405951377704, 1.000000000000000000, 0.9876883405951377704, 1.000000000000000000, 0.9876883405951377704, 1.000000000000000000, 0.9876883405951377704, 1.000000000000000000, 0.9876883405951377704, 1.000000000000000000),
 ( 1.000000000000000000, 0.9876883405951377704, 1.000000000000000000, 0.9876883405951377704, 1.000000000000000000, 0.9876883405951377704, 1.000000000000000000, 0.9876883405951377704, 1.000000000000000000, 0.9876883405951377704, 1.000000000000000000, 0.9876883405951377704, 1.000000000000000000, 0.9876883405951377704, 1.000000000000000000, 0.9876883405951377704, 1.000000000000000000) ) ) 
 REPRESENTATION_ITEM ( '' )  SURFACE ( )  );
#6161=CARTESIAN_POINT ( 'NONE',  ( 4.611396867937178179, -3.350375938067129855, -9.312499995903225525 ) ) ;
#6171=CARTESIAN_POINT ( 'NONE',  ( -5.700000000000000178, -2.180340287075187351E-16, -12.66727757604271076 ) ) ;
#6174=CARTESIAN_POINT ( 'NONE',  ( 3.499494075959815653, 3.499494075959816541, -13.96874999795161365 ) ) ;
#6178=VERTEX_POINT ( 'NONE', #1195 ) ;
#6188=FACE_BOUND ( 'NONE', #3936, .T. ) ;
#6192=CARTESIAN_POINT ( 'NONE',  ( 3.814044456245474279, -4.235925505221167064, -12.00000000000000533 ) ) ;
#6205=CARTESIAN_POINT ( 'NONE',  ( -5.700000000000001066, 0.000000000000000000, -6.656249997951614539 ) ) ;
#6212=CARTESIAN_POINT ( 'NONE',  ( 4.484949146646356688, -3.631840208645826351, -12.81249999590322552 ) ) ;
#6214=EDGE_CURVE ( 'NONE', #13293, #16711, #8333, .T. ) ;
#6230=DIRECTION ( 'NONE',  ( 1.000000000000000000, 0.000000000000000000, 0.000000000000000000 ) ) ;
#6263=CARTESIAN_POINT ( 'NONE',  ( 1.185096637661176677, -5.575441324182703440, -8.312499995903225525 ) ) ;
#6267=CARTESIAN_POINT ( 'NONE',  ( 4.080749450109649956, 4.080749450109650844, -13.50000000000000533 ) ) ;
#6287=CARTESIAN_POINT ( 'NONE',  ( 3.143139765844590983, -4.840010801796506001, -12.50000000000000533 ) ) ;
#6314=CARTESIAN_POINT ( 'NONE',  ( 3.114526743279282694, 3.846120219227923798, -6.968749997951614539 ) ) ;
#6316=CARTESIAN_POINT ( 'NONE',  ( 1.280903732194421663, -4.780397808154265960, -13.96874999795161365 ) ) ;
#6321=VERTEX_POINT ( 'NONE', #11186 ) ;
#6338=CARTESIAN_POINT ( 'NONE',  ( 2.695436003842732298, 4.150607464521792522, -10.34374999795161543 ) ) ;
#6357=CARTESIAN_POINT ( 'NONE',  ( -5.574407415329146964, 1.493657965219562067, -13.50000000000000533 ) ) ;
#6359=CARTESIAN_POINT ( 'NONE',  ( -4.781284448697179279, 1.016293382781477961, -10.84374999795161543 ) ) ;
#6375=DIRECTION ( 'NONE',  ( 1.000000000000000000, 0.000000000000000000, 0.000000000000000000 ) ) ;
#6378=LINE ( 'NONE', #12507, #2643 ) ;
#6408=CARTESIAN_POINT ( 'NONE',  ( 4.780397808154266848, 1.280903732194421218, -9.343749997951615427 ) ) ;
#6441=CARTESIAN_POINT ( 'NONE',  ( -0.5958122406256771697, -5.668774803599153422, -8.000000000000005329 ) ) ;
#6451=CARTESIAN_POINT ( 'NONE',  ( -4.484949146646406426, -3.631840208645764179, -11.81249999590322552 ) ) ;
#6455=CARTESIAN_POINT ( 'NONE',  ( -2.620002426024544473, 5.142044285764749922, -9.500000000000003553 ) ) ;
#6460=ORIENTED_EDGE ( 'NONE', *, *, #14395, .T. ) ;
#6467=CARTESIAN_POINT ( 'NONE',  ( 4.648860486681943627, -1.510506337161893864, -7.468749997951615427 ) ) ;
#6471=SHAPE_REPRESENTATION_RELATIONSHIP ( 'NONE' , 'NONE' ,  #6040, #9489 ) ;
#6472=DIRECTION ( 'NONE',  ( 1.000000000000000000, 0.000000000000000000, 0.000000000000000000 ) ) ;
#6500=CARTESIAN_POINT ( 'NONE',  ( 1.510506337161861223, 4.648860486681953397, -12.46874999795161543 ) ) ;
#6507=CARTESIAN_POINT ( 'NONE',  ( 0.000000000000000000, 0.000000000000000000, -18.00000000000000355 ) ) ;
#6511=CARTESIAN_POINT ( 'NONE',  ( 4.233219804643871598, -2.444050593750019651, -11.46874999795161543 ) ) ;
#6525=ORIENTED_EDGE ( 'NONE', *, *, #7556, .T. ) ;
#6534=ORIENTED_EDGE ( 'NONE', *, *, #3700, .T. ) ;
#6550=VERTEX_POINT ( 'NONE', #17748 ) ;
#6551=CARTESIAN_POINT ( 'NONE',  ( -3.114526743279308896, -3.846120219227901149, -6.968749997951614539 ) ) ;
#6556=CARTESIAN_POINT ( 'NONE',  ( -3.954556930911862000, 2.873153789725825469, -8.468749997951615427 ) ) ;
#6561=ORIENTED_EDGE ( 'NONE', *, *, #838, .T. ) ;
#6572=DIRECTION ( 'NONE',  ( 0.6363829547955638377, 7.793443486223220387E-17, -0.7713732785400770897 ) ) ;
#6573=CARTESIAN_POINT ( 'NONE',  ( 3.143139765844622957, 4.840010801796482909, -10.81249999590322375 ) ) ;
#6576=PRODUCT_DEFINITION_CONTEXT ( 'detailed design', #7767, 'design' ) ;
#6579=CARTESIAN_POINT ( 'NONE',  ( 0.5109457054261454800, -4.861323657744410554, -14.46874999795161720 ) ) ;
#6581=CARTESIAN_POINT ( 'NONE',  ( 5.574407415329157622, -1.493657965219523209, -14.81249999590322375 ) ) ;
#6590=EDGE_CURVE ( 'NONE', #1462, #5861, #3945, .T. ) ;
#6593=EDGE_CURVE ( 'NONE', #11735, #1617, #14756, .T. ) ;
#6598=CARTESIAN_POINT ( 'NONE',  ( 2.873153789725825025, 3.954556930911862000, -13.46874999795161543 ) ) ;
#6615=CARTESIAN_POINT ( 'NONE',  ( 3.954556930911861112, 2.873153789725825913, -14.84374999795161543 ) ) ;
#6618=CARTESIAN_POINT ( 'NONE',  ( -4.465502636338010589, 1.988169868018623720, -14.46874999795161720 ) ) ;
#6625=CARTESIAN_POINT ( 'NONE',  ( -5.700000000000001066, 1.090170143537592985E-15, -10.64522241986045259 ) ) ;
#6643=CARTESIAN_POINT ( 'NONE',  ( -3.143139765844656264, -4.840010801796461593, -9.500000000000005329 ) ) ;
#6673=( LENGTH_UNIT ( ) NAMED_UNIT ( * ) SI_UNIT ( .MILLI., .METRE. ) );
#6676=( BOUNDED_SURFACE ( )  B_SPLINE_SURFACE ( 1, 2, ( 
 ( #19723, #7709, #5911, #6007, #1615, #19626, #4618, #10433, #12128, #18233, #9024, #13723, #12, #16933, #9126, #16535, #18133 ),
 ( #4511, #13825, #15231, #2811, #1524, #7399, #15428, #10528, #7609, #19518, #16625, #9324, #18327, #13523, #12029, #18422, #3210 ) ),
 .UNSPECIFIED., .F., .F., .T. ) 
 B_SPLINE_SURFACE_WITH_KNOTS ( ( 2, 2 ),
 ( 3, 2, 2, 2, 2, 2, 2, 2, 3 ),
 ( 0.000000000000000000, 1.000000000000000000 ),
 ( 0.000000000000000000, 0.05000000000000000278, 0.1000000000000000056, 0.1499999999999999944, 0.2000000000000000111, 0.2500000000000000000, 0.2999999999999999889, 0.3499999999999999778, 0.4000000000000000222 ),
 .UNSPECIFIED. ) 
 GEOMETRIC_REPRESENTATION_ITEM ( )  RATIONAL_B_SPLINE_SURFACE ( (
 ( 1.000000000000000000, 0.9876883405951377704, 1.000000000000000000, 0.9876883405951377704, 1.000000000000000000, 0.9876883405951377704, 1.000000000000000000, 0.9876883405951377704, 1.000000000000000000, 0.9876883405951377704, 1.000000000000000000, 0.9876883405951377704, 1.000000000000000000, 0.9876883405951377704, 1.000000000000000000, 0.9876883405951377704, 1.000000000000000000),
 ( 1.000000000000000000, 0.9876883405951377704, 1.000000000000000000, 0.9876883405951377704, 1.000000000000000000, 0.9876883405951377704, 1.000000000000000000, 0.9876883405951377704, 1.000000000000000000, 0.9876883405951377704, 1.000000000000000000, 0.9876883405951377704, 1.000000000000000000, 0.9876883405951377704, 1.000000000000000000, 0.9876883405951377704, 1.000000000000000000) ) ) 
 REPRESENTATION_ITEM ( '' )  SURFACE ( )  );
#6679=CARTESIAN_POINT ( 'NONE',  ( 3.846120219227923798, -3.114526743279282250, -12.34374999795161543 ) ) ;
#6684=CARTESIAN_POINT ( 'NONE',  ( -4.888101187500000222, 0.000000000000000000, -6.843749997951615427 ) ) ;
#6704=ORIENTED_EDGE ( 'NONE', *, *, #7324, .T. ) ;
#6709=CARTESIAN_POINT ( 'NONE',  ( 3.846120219227923798, -3.114526743279282250, -12.34374999795161543 ) ) ;
#6718=CARTESIAN_POINT ( 'NONE',  ( 1.016293382781377819, -4.781284448697200595, -7.468749997951615427 ) ) ;
#6721=CARTESIAN_POINT ( 'NONE',  ( 1.510506337161829027, -4.648860486681964055, -10.46874999795161720 ) ) ;
#6745=CARTESIAN_POINT ( 'NONE',  ( -4.620319390059805187, 1.773574444220790136, -10.96874999795161720 ) ) ;
#6755=CARTESIAN_POINT ( 'NONE',  ( 5.207209108562820710, -2.318398865532073305, -14.00000000000000533 ) ) ;
#6767=AXIS2_PLACEMENT_3D ( 'NONE', #598, #502, #6375 ) ;
#6773=CIRCLE ( 'NONE', #9354, 5.700000000000001954 ) ;
#6780=UNCERTAINTY_MEASURE_WITH_UNIT (LENGTH_MEASURE( 1.000000000000000082E-05 ), #9507, 'distance_accuracy_value', 'NONE');
#6785=CARTESIAN_POINT ( 'NONE',  ( -1.280903732194487166, -4.780397808154247308, -9.343749997951615427 ) ) ;
#6796=( BOUNDED_CURVE ( )  B_SPLINE_CURVE ( 2, ( #1824, #532, #12434, #14030, #18628, #6212, #5020, #9742, #4726, #11131, #17231 ),
 .UNSPECIFIED., .F., .F. ) 
 B_SPLINE_CURVE_WITH_KNOTS ( ( 3, 2, 2, 2, 2, 3 ),
 ( 0.1666819079834116757, 0.2000000000000000111, 0.2500000000000000000, 0.2999999999999999889, 0.3499999999999999778, 0.4000000000000000222 ),
 .UNSPECIFIED. ) 
 CURVE ( )  GEOMETRIC_REPRESENTATION_ITEM ( )  RATIONAL_B_SPLINE_CURVE ( ( 0.9945256517182512468, 0.9917959799814380917, 1.000000000000000000, 0.9876883405951377704, 1.000000000000000000, 0.9876883405951377704, 1.000000000000000000, 0.9876883405951377704, 1.000000000000000000, 0.9876883405951377704, 1.000000000000000000 ) ) 
 REPRESENTATION_ITEM ( '' )  );
#6801=EDGE_CURVE ( 'NONE', #15763, #488, #5824, .T. ) ;
#6809=CARTESIAN_POINT ( 'NONE',  ( -2.620002426024544473, 5.142044285764750811, -10.81249999590322375 ) ) ;
#6811=CARTESIAN_POINT ( 'NONE',  ( -3.490243377569957047E-16, 5.700000000000001066, -11.00000000000000711 ) ) ;
#6822=CARTESIAN_POINT ( 'NONE',  ( 1.761396867937162769, -5.421022142882388373, -11.31249999590322375 ) ) ;
#6852=CARTESIAN_POINT ( 'NONE',  ( -5.387740456496206143, 2.068159791354259092, -10.50000000000000711 ) ) ;
#6869=CARTESIAN_POINT ( 'NONE',  ( -2.849999999999989431, 4.936344801571308061, -6.656249997951614539 ) ) ;
#6871=CARTESIAN_POINT ( 'NONE',  ( 5.575441324182695446, 1.185096637661216201, -13.31249999590322730 ) ) ;
#6880=CARTESIAN_POINT ( 'NONE',  ( 0.2590123213420630899, -4.942249507334558700, -8.343749997951613651 ) ) ;
#6912=ADVANCED_FACE ( 'NONE', ( #18928 ), #17965, .T. ) ;
#6913=( BOUNDED_CURVE ( )  B_SPLINE_CURVE ( 2, ( #7481, #4592, #16605, #12198, #13698 ),
 .UNSPECIFIED., .F., .F. ) 
 B_SPLINE_CURVE_WITH_KNOTS ( ( 3, 2, 3 ),
 ( 0.3333180920165860761, 0.3499999999999999778, 0.4000000000000000222 ),
 .UNSPECIFIED. ) 
 CURVE ( )  GEOMETRIC_REPRESENTATION_ITEM ( )  RATIONAL_B_SPLINE_CURVE ( ( 0.9945256517182510247, 0.9958923606136991236, 1.000000000000000000, 0.9876883405951377704, 1.000000000000000000 ) ) 
 REPRESENTATION_ITEM ( '' )  );
#6914=B_SPLINE_CURVE_WITH_KNOTS ( 'NONE', 1,
 ( #12174, #4961 ),
 .UNSPECIFIED., .F., .F.,
 ( 2, 2 ),
 ( 0.000000000000000000, 1.000000000000000000 ),
 .UNSPECIFIED. ) ;
#6919=CARTESIAN_POINT ( 'NONE',  ( 4.611396867937178179, -3.350375938067129855, -9.312499995903225525 ) ) ;
#6932=FACE_OUTER_BOUND ( 'NONE', #18768, .T. ) ;
#6936=AXIS2_PLACEMENT_3D ( 'NONE', #12665, #8646, #8846 ) ;
#6937=ORIENTED_EDGE ( 'NONE', *, *, #15988, .F. ) ;
#6944=ORIENTED_EDGE ( 'NONE', *, *, #4890, .F. ) ;
#6970=ORIENTED_EDGE ( 'NONE', *, *, #11649, .T. ) ;
#6972=CARTESIAN_POINT ( 'NONE',  ( -4.465502636338010589, 1.988169868018623720, -14.46874999795161720 ) ) ;
#6974=CARTESIAN_POINT ( 'NONE',  ( 0.5109457054261454800, -4.861323657744410554, -14.84374999795161543 ) ) ;
#6985=DIRECTION ( 'NONE',  ( -0.000000000000000000, -0.000000000000000000, 1.000000000000000000 ) ) ;
#6988=DIRECTION ( 'NONE',  ( -0.8660254037844399289, -0.4999999999999978906, 0.000000000000000000 ) ) ;
#6993=CARTESIAN_POINT ( 'NONE',  ( -2.849999999999988987, 4.936344801571308061, -6.000000000000005329 ) ) ;
#7008=EDGE_CURVE ( 'NONE', #2089, #8012, #9770, .T. ) ;
#7025=DIRECTION ( 'NONE',  ( 1.000000000000000000, 0.000000000000000000, 0.000000000000000000 ) ) ;
#7028=( BOUNDED_CURVE ( )  B_SPLINE_CURVE ( 2, ( #16864, #12260, #4356, #18066, #18359, #13449, #14962, #8957, #19752, #4653, #7537, #9060, #15265, #3147, #18168, #19551, #1158 ),
 .UNSPECIFIED., .F., .F. ) 
 B_SPLINE_CURVE_WITH_KNOTS ( ( 3, 2, 2, 2, 2, 2, 2, 2, 3 ),
 ( 0.000000000000000000, 0.05000000000000000971, 0.1000000000000000194, 0.1499999999999999944, 0.2000000000000000389, 0.2500000000000000000, 0.2999999999999999889, 0.3499999999999999223, 0.4000000000000000777 ),
 .UNSPECIFIED. ) 
 CURVE ( )  GEOMETRIC_REPRESENTATION_ITEM ( )  RATIONAL_B_SPLINE_CURVE ( ( 1.000000000000000000, 0.9876883405951377704, 1.000000000000000000, 0.9876883405951377704, 1.000000000000000000, 0.9876883405951377704, 1.000000000000000000, 0.9876883405951377704, 1.000000000000000000, 0.9876883405951377704, 1.000000000000000000, 0.9876883405951377704, 1.000000000000000000, 0.9876883405951377704, 1.000000000000000000, 0.9876883405951377704, 1.000000000000000000 ) ) 
 REPRESENTATION_ITEM ( '' )  );
#7031=DIRECTION ( 'NONE',  ( -0.8660254037844398178, 0.000000000000000000, 0.4999999999999979461 ) ) ;
#7036=CARTESIAN_POINT ( 'NONE',  ( -3.632567103900569361, -3.270778111535287191, -7.843749997951614539 ) ) ;
#7044=ORIENTED_EDGE ( 'NONE', *, *, #12130, .T. ) ;
#7055=B_SPLINE_CURVE_WITH_KNOTS ( 'NONE', 1,
 ( #5761, #7456 ),
 .UNSPECIFIED., .F., .F.,
 ( 2, 2 ),
 ( 0.000000000000000000, 1.000000000000000000 ),
 .UNSPECIFIED. ) ;
#7059=DIRECTION ( 'NONE',  ( -0.000000000000000000, -0.000000000000000000, 1.000000000000000000 ) ) ;
#7068=CARTESIAN_POINT ( 'NONE',  ( 3.270778111535314281, -3.632567103900546712, -12.46874999795161543 ) ) ;
#7069=ORIENTED_EDGE ( 'NONE', *, *, #134, .T. ) ;
#7071=AXIS2_PLACEMENT_3D ( 'NONE', #4898, #11301, #6472 ) ;
#7072=CARTESIAN_POINT ( 'NONE',  ( 4.840010801796506001, 3.143139765844590983, -8.812499995903225525 ) ) ;
#7073=EDGE_LOOP ( 'NONE', ( #3190, #3777, #3593, #6944 ) ) ;
#7087=EDGE_LOOP ( 'NONE', ( #10963, #15149, #15037, #9160 ) ) ;
#7095=CARTESIAN_POINT ( 'NONE',  ( 4.080749450109649956, 4.080749450109650844, -13.50000000000000533 ) ) ;
#7110=CARTESIAN_POINT ( 'NONE',  ( -1.761396867937238042, -5.421022142882365280, -12.00000000000000533 ) ) ;
#7123=CARTESIAN_POINT ( 'NONE',  ( -0.7741991708319226895, -4.888101187499994893, -12.34374999795161543 ) ) ;
#7138=FACE_OUTER_BOUND ( 'NONE', #2194, .T. ) ;
#7158=CARTESIAN_POINT ( 'NONE',  ( 0.000000000000000000, 0.000000000000000000, 0.000000000000000000 ) ) ;
#7166=CARTESIAN_POINT ( 'NONE',  ( -1.493657965219446160, 5.574407415329178939, -13.50000000000000533 ) ) ;
#7168=CARTESIAN_POINT ( 'NONE',  ( -4.888101187500000222, 0.7741991708318887166, -7.343749997951615427 ) ) ;
#7185=EDGE_LOOP ( 'NONE', ( #19751, #15862, #8968, #798 ) ) ;
#7191=EDGE_CURVE ( 'NONE', #9505, #19556, #10717, .T. ) ;
#7193=CARTESIAN_POINT ( 'NONE',  ( -1.761396867937200739, 5.421022142882375938, -10.00000000000000533 ) ) ;
#7201=CARTESIAN_POINT ( 'NONE',  ( 5.142044285764733935, -2.620002426024580000, -8.812499995903225525 ) ) ;
#7229=ORIENTED_EDGE ( 'NONE', *, *, #5542, .F. ) ;
#7232=CARTESIAN_POINT ( 'NONE',  ( 0.2590123213420631454, -4.942249507334558700, -7.968749997951616315 ) ) ;
#7234=CARTESIAN_POINT ( 'NONE',  ( 3.814044456245502701, 4.235925505221138643, -11.31249999590322375 ) ) ;
#7281=CARTESIAN_POINT ( 'NONE',  ( 1.280903732194421440, -4.780397808154265071, -14.34374999795161543 ) ) ;
#7287=ADVANCED_FACE ( 'NONE', ( #17308 ), #10014, .T. ) ;
#7302=CARTESIAN_POINT ( 'NONE',  ( -1.016293382781411125, 4.781284448697194378, -7.468749997951615427 ) ) ;
#7309=EDGE_LOOP ( 'NONE', ( #19719, #4355, #7924, #6009 ) ) ;
#7311=( LENGTH_UNIT ( ) NAMED_UNIT ( * ) SI_UNIT ( .MILLI., .METRE. ) );
#7315=CARTESIAN_POINT ( 'NONE',  ( 1.510506337161829027, -4.648860486681964055, -10.46874999795161720 ) ) ;
#7324=EDGE_CURVE ( 'NONE', #4661, #5399, #18441, .T. ) ;
#7325=PRODUCT_DEFINITION ( 'UNKNOWN', '', #14993, #6576 ) ;
#7332=CARTESIAN_POINT ( 'NONE',  ( -1.280903732194487166, -4.780397808154247308, -8.968749997951611874 ) ) ;
#7339=VECTOR ( 'NONE', #14077, 1000.000000000000000 ) ;
#7343=CARTESIAN_POINT ( 'NONE',  ( 4.484949146646379781, 3.631840208645794821, -10.50000000000000533 ) ) ;
#7354=CARTESIAN_POINT ( 'NONE',  ( 3.350375938067065462, -4.611396867937225252, -10.31249999590322552 ) ) ;
#7362=CARTESIAN_POINT ( 'NONE',  ( -4.484949146646330931, 3.631840208645857437, -11.50000000000000355 ) ) ;
#7365=CARTESIAN_POINT ( 'NONE',  ( -5.207209108562852684, -2.318398865532001363, -9.312499995903225525 ) ) ;
#7376=ORIENTED_EDGE ( 'NONE', *, *, #18316, .T. ) ;
#7386=CYLINDRICAL_SURFACE ( 'NONE', #17902, 4.200000000000001066 ) ;
#7399=CARTESIAN_POINT ( 'NONE',  ( -3.499494075959816541, 3.499494075959816541, -8.968749997951611874 ) ) ;
#7402=CARTESIAN_POINT ( 'NONE',  ( 3.846120219227944670, 3.114526743279255161, -11.34374999795161543 ) ) ;
#7418=EDGE_LOOP ( 'NONE', ( #12926, #2066, #14352, #1050 ) ) ;
#7421=FACE_OUTER_BOUND ( 'NONE', #7087, .T. ) ;
#7430=CARTESIAN_POINT ( 'NONE',  ( 4.484949146646356688, -3.631840208645826351, -11.50000000000000355 ) ) ;
#7437=CARTESIAN_POINT ( 'NONE',  ( 2.444050593749960587, -4.233219804643904460, -6.468749997951615427 ) ) ;
#7438=CARTESIAN_POINT ( 'NONE',  ( 1.185096637661176677, -5.575441324182703440, -8.312499995903225525 ) ) ;
#7442=CARTESIAN_POINT ( 'NONE',  ( 5.387740456496232788, 2.068159791354184485, -12.81249999590322552 ) ) ;
#7456=CARTESIAN_POINT ( 'NONE',  ( -5.207209108562804722, 2.318398865532109276, -15.31249999590322552 ) ) ;
#7458=CARTESIAN_POINT ( 'NONE',  ( 4.080749450109622423, -4.080749450109678378, -9.812499995903225525 ) ) ;
#7468=CARTESIAN_POINT ( 'NONE',  ( -4.936344801571268093, 2.850000000000057820, -11.00000000000000711 ) ) ;
#7472=CARTESIAN_POINT ( 'NONE',  ( 3.954556930911861112, 2.873153789725825913, -14.84374999795161543 ) ) ;
#7476=CARTESIAN_POINT ( 'NONE',  ( -3.846120219227901149, 3.114526743279308896, -11.96874999795161365 ) ) ;
#7481=CARTESIAN_POINT ( 'NONE',  ( -5.700000000000000178, -2.180340287075187351E-16, -13.97977757194593273 ) ) ;
#7497=CARTESIAN_POINT ( 'NONE',  ( 1.280903732194454081, 4.780397808154257078, -9.343749997951615427 ) ) ;
#7498=EDGE_CURVE ( 'NONE', #17369, #5524, #684, .T. ) ;
#7505=LINE ( 'NONE', #6205, #1820 ) ;
#7509=CARTESIAN_POINT ( 'NONE',  ( -4.648860486681953397, 1.510506337161861445, -7.468749997951615427 ) ) ;
#7523=ORIENTED_EDGE ( 'NONE', *, *, #12236, .F. ) ;
#7527=ORIENTED_EDGE ( 'NONE', *, *, #18445, .F. ) ;
#7534=CARTESIAN_POINT ( 'NONE',  ( 3.631840208645826795, 4.484949146646356688, -6.500000000000005329 ) ) ;
#7537=CARTESIAN_POINT ( 'NONE',  ( 4.233219804643887585, 2.444050593749990785, -11.46874999795161543 ) ) ;
#7546=CARTESIAN_POINT ( 'NONE',  ( 5.207209108562820710, -2.318398865532073305, -15.31249999590322552 ) ) ;
#7553=ORIENTED_EDGE ( 'NONE', *, *, #16459, .T. ) ;
#7556=EDGE_CURVE ( 'NONE', #11278, #5399, #3297, .T. ) ;
#7609=CARTESIAN_POINT ( 'NONE',  ( -1.510506337161861667, 4.648860486681953397, -10.46874999795161720 ) ) ;
#7618=VECTOR ( 'NONE', #9142, 1000.000000000000227 ) ;
#7619=DIRECTION ( 'NONE',  ( -1.000000000000000000, 6.982962677686267499E-15, 0.000000000000000000 ) ) ;
#7629=B_SPLINE_CURVE_WITH_KNOTS ( 'NONE', 1,
 ( #1978, #7976 ),
 .UNSPECIFIED., .F., .F.,
 ( 2, 2 ),
 ( 0.000000000000000000, 1.000000000000000000 ),
 .UNSPECIFIED. ) ;
#7630=B_SPLINE_CURVE_WITH_KNOTS ( 'NONE', 1,
 ( #1022, #2517 ),
 .UNSPECIFIED., .F., .F.,
 ( 2, 2 ),
 ( 0.000000000000000000, 1.000000000000000000 ),
 .UNSPECIFIED. ) ;
#7638=CIRCLE ( 'NONE', #18832, 5.700000000000001954 ) ;
#7639=CARTESIAN_POINT ( 'NONE',  ( 5.207209108562838473, 2.318398865532038666, -8.000000000000005329 ) ) ;
#7676=( BOUNDED_CURVE ( )  B_SPLINE_CURVE ( 2, ( #1025, #14836, #5616, #1130, #13421, #19521, #386, #3683, #5082 ),
 .UNSPECIFIED., .F., .F. ) 
 B_SPLINE_CURVE_WITH_KNOTS ( ( 3, 2, 2, 2, 3 ),
 ( 0.000000000000000000, 0.04999999999999999584, 0.09999999999999999167, 0.1499999999999999944, 0.1666819079834116757 ),
 .UNSPECIFIED. ) 
 CURVE ( )  GEOMETRIC_REPRESENTATION_ITEM ( )  RATIONAL_B_SPLINE_CURVE ( ( 1.000000000000000000, 0.9876883405951377704, 1.000000000000000000, 0.9876883405951377704, 1.000000000000000000, 0.9876883405951377704, 1.000000000000000000, 0.9958923606136996787, 0.9945256517182512468 ) ) 
 REPRESENTATION_ITEM ( '' )  );
#7678=AXIS2_PLACEMENT_3D ( 'NONE', #5402, #13109, #906 ) ;
#7695=CARTESIAN_POINT ( 'NONE',  ( 4.936344801571289409, -2.850000000000023626, -11.00000000000000711 ) ) ;
#7698=DIRECTION ( 'NONE',  ( -0.000000000000000000, -0.000000000000000000, 1.000000000000000000 ) ) ;
#7709=CARTESIAN_POINT ( 'NONE',  ( -4.888101187500000222, 0.7741991708318887166, -7.343749997951615427 ) ) ;
#7728=DIRECTION ( 'NONE',  ( -1.000000000000000000, 0.000000000000000000, 0.000000000000000000 ) ) ;
#7745=DIRECTION ( 'NONE',  ( -0.000000000000000000, -0.000000000000000000, 1.000000000000000000 ) ) ;
#7749=CARTESIAN_POINT ( 'NONE',  ( -2.318398865532109721, -5.207209108562803834, -10.31249999590322552 ) ) ;
#7754=CARTESIAN_POINT ( 'NONE',  ( 2.849999999999954348, -4.936344801571327601, -6.656249997951614539 ) ) ;
#7761=VECTOR ( 'NONE', #10849, 1000.000000000000000 ) ;
#7767=APPLICATION_CONTEXT ( 'automotive_design' ) ;
#7774=CARTESIAN_POINT ( 'NONE',  ( 2.849999999999954348, -4.936344801571327601, -7.312499995903225525 ) ) ;
#7778=CARTESIAN_POINT ( 'NONE',  ( 1.761396867937200073, 5.421022142882376826, -12.00000000000000533 ) ) ;
#7788=CARTESIAN_POINT ( 'NONE',  ( -5.207209108562852684, -2.318398865532001363, -9.312499995903225525 ) ) ;
#7795=CARTESIAN_POINT ( 'NONE',  ( 5.700000000000001066, -0.2987243419133416289, -12.83455515208547304 ) ) ;
#7802=CARTESIAN_POINT ( 'NONE',  ( -3.499494075959816541, 3.499494075959816541, -9.343749997951615427 ) ) ;
#7830=DIRECTION ( 'NONE',  ( 0.5877852522924679191, -0.8090169943749512260, 0.000000000000000000 ) ) ;
#7839=VERTEX_POINT ( 'NONE', #5163 ) ;
#7848=CARTESIAN_POINT ( 'NONE',  ( 5.575441324182695446, 1.185096637661216201, -13.31249999590322730 ) ) ;
#7856=CARTESIAN_POINT ( 'NONE',  ( -3.814044456245531567, -4.235925505221111997, -10.00000000000000533 ) ) ;
#7870=CARTESIAN_POINT ( 'NONE',  ( -3.490243377569957047E-16, 5.700000000000001066, -11.00000000000000711 ) ) ;
#7880=CARTESIAN_POINT ( 'NONE',  ( -5.700000000000001066, 1.090170143537592985E-15, -10.64522241986045259 ) ) ;
#7883=ORIENTED_EDGE ( 'NONE', *, *, #16920, .T. ) ;
#7910=CARTESIAN_POINT ( 'NONE',  ( -0.7741991708318890497, 4.888101187500000222, -10.96874999795161720 ) ) ;
#7922=CARTESIAN_POINT ( 'NONE',  ( -5.700000000000001066, 0.000000000000000000, -6.000000000000005329 ) ) ;
#7924=ORIENTED_EDGE ( 'NONE', *, *, #15785, .F. ) ;
#7965=CARTESIAN_POINT ( 'NONE',  ( 2.647025296874957689, -4.584782303107616031, -6.234374998975811266 ) ) ;
#7971=CARTESIAN_POINT ( 'NONE',  ( -5.421022142882375938, 1.761396867937200517, -7.000000000000005329 ) ) ;
#7972=ORIENTED_EDGE ( 'NONE', *, *, #615, .T. ) ;
#7976=CARTESIAN_POINT ( 'NONE',  ( 4.465502636338025688, -1.988169868018592856, -14.46874999795161720 ) ) ;
#7982=LINE ( 'NONE', #3583, #2658 ) ;
#7986=( NAMED_UNIT ( * ) SI_UNIT ( $, .STERADIAN. ) SOLID_ANGLE_UNIT ( ) );
#7989=ORIENTED_EDGE ( 'NONE', *, *, #12130, .F. ) ;
#7994=CARTESIAN_POINT ( 'NONE',  ( -2.850000000000058265, -4.936344801571268093, -6.000000000000005329 ) ) ;
#8009=CARTESIAN_POINT ( 'NONE',  ( -2.993098736590125853E-16, 4.888101187500000222, -11.46874999795161543 ) ) ;
#8012=VERTEX_POINT ( 'NONE', #2830 ) ;
#8016=CARTESIAN_POINT ( 'NONE',  ( 0.2590123213420631454, -4.942249507334558700, -8.343749997951611874 ) ) ;
#8018=CARTESIAN_POINT ( 'NONE',  ( 4.465502636338039011, 1.988169868018562436, -8.468749997951615427 ) ) ;
#8036=ORIENTED_EDGE ( 'NONE', *, *, #790, .T. ) ;
#8039=PLANE ( 'NONE',  #19506 ) ;
#8042=VERTEX_POINT ( 'NONE', #234 ) ;
#8045=ORIENTED_EDGE ( 'NONE', *, *, #13728, .F. ) ;
#8047=CARTESIAN_POINT ( 'NONE',  ( -4.150607464521828938, -2.695436003842674122, -8.343749997951613651 ) ) ;
#8063=ADVANCED_FACE ( 'NONE', ( #15545 ), #3230, .T. ) ;
#8072=CARTESIAN_POINT ( 'NONE',  ( 2.873153789725825025, 3.954556930911862000, -13.46874999795161543 ) ) ;
#8085=CARTESIAN_POINT ( 'NONE',  ( 4.465502636338025688, -1.988169868018592412, -14.84374999795161543 ) ) ;
#8086=( NAMED_UNIT ( * ) PLANE_ANGLE_UNIT ( ) SI_UNIT ( $, .RADIAN. ) );
#8089=CARTESIAN_POINT ( 'NONE',  ( 5.700000000000001066, 0.000000000000000000, -13.97977757194595760 ) ) ;
#8094=ADVANCED_FACE ( 'NONE', ( #10745 ), #18265, .T. ) ;
#8095=CARTESIAN_POINT ( 'NONE',  ( 4.484949146646356688, -3.631840208645826351, -11.50000000000000355 ) ) ;
#8100=COLOUR_RGB ( '', 0.31764706, 0.68627451, 0.89019608) ;
#8106=DIRECTION ( 'NONE',  ( 1.000000000000000000, 0.000000000000000000, 0.000000000000000000 ) ) ;
#8126=CARTESIAN_POINT ( 'NONE',  ( -4.781284448697201483, -1.016293382781378485, -12.84374999795161543 ) ) ;
#8176=FACE_OUTER_BOUND ( 'NONE', #1099, .T. ) ;
#8177=ORIENTED_EDGE ( 'NONE', *, *, #10519, .F. ) ;
#8192=CARTESIAN_POINT ( 'NONE',  ( 4.936344801571308061, 2.849999999999989875, -12.31249999590322552 ) ) ;
#8216=CARTESIAN_POINT ( 'NONE',  ( -4.484949146646330931, 3.631840208645857437, -12.81249999590322552 ) ) ;
#8223=ADVANCED_FACE ( 'NONE', ( #17442 ), #805, .T. ) ;
#8242=CARTESIAN_POINT ( 'NONE',  ( 4.409619785863891472, -2.246813503491864150, -7.968749997951616315 ) ) ;
#8252=ORIENTED_EDGE ( 'NONE', *, *, #7556, .F. ) ;
#8259=CARTESIAN_POINT ( 'NONE',  ( -4.233219804643852946, 2.444050593750049405, -11.84374999795161365 ) ) ;
#8269=DIRECTION ( 'NONE',  ( -0.4330127018922130255, 0.7500000000000049960, 0.4999999999999980571 ) ) ;
#8271=ORIENTED_EDGE ( 'NONE', *, *, #9164, .T. ) ;
#8272=CARTESIAN_POINT ( 'NONE',  ( -4.840010801796527318, -3.143139765844555900, -7.500000000000005329 ) ) ;
#8287=CARTESIAN_POINT ( 'NONE',  ( -3.350375938067128967, -4.611396867937178179, -13.00000000000000533 ) ) ;
#8296=CARTESIAN_POINT ( 'NONE',  ( 2.695436003842704764, -4.150607464521812062, -13.34374999795161365 ) ) ;
#8300=CARTESIAN_POINT ( 'NONE',  ( -0.5745956068256975469, 5.466912017135477697, -14.11718749948790830 ) ) ;
#8301=CARTESIAN_POINT ( 'NONE',  ( -0.5109457054262123155, -4.861323657744403448, -8.843749997951615427 ) ) ;
#8315=CARTESIAN_POINT ( 'NONE',  ( 3.499494075959815653, 3.499494075959816541, -13.96874999795161365 ) ) ;
#8322=VECTOR ( 'NONE', #6088, 1000.000000000000000 ) ;
#8333=( BOUNDED_CURVE ( )  B_SPLINE_CURVE ( 2, ( #16503, #4391, #10503, #2781, #14999, #8897, #8996, #1291, #16601, #15100, #1396, #7476, #13595, #19693, #5977, #12100, #15198 ),
 .UNSPECIFIED., .F., .F. ) 
 B_SPLINE_CURVE_WITH_KNOTS ( ( 3, 2, 2, 2, 2, 2, 2, 2, 3 ),
 ( 0.000000000000000000, 0.05000000000000000971, 0.1000000000000000194, 0.1499999999999999944, 0.2000000000000000389, 0.2500000000000000000, 0.2999999999999999889, 0.3499999999999999223, 0.4000000000000000777 ),
 .UNSPECIFIED. ) 
 CURVE ( )  GEOMETRIC_REPRESENTATION_ITEM ( )  RATIONAL_B_SPLINE_CURVE ( ( 1.000000000000000000, 0.9876883405951377704, 1.000000000000000000, 0.9876883405951377704, 1.000000000000000000, 0.9876883405951377704, 1.000000000000000000, 0.9876883405951377704, 1.000000000000000000, 0.9876883405951377704, 1.000000000000000000, 0.9876883405951377704, 1.000000000000000000, 0.9876883405951377704, 1.000000000000000000, 0.9876883405951377704, 1.000000000000000000 ) ) 
 REPRESENTATION_ITEM ( '' )  );
#8338=CARTESIAN_POINT ( 'NONE',  ( -4.780397808154247308, 1.280903732194486722, -13.96874999795161365 ) ) ;
#8341=DIRECTION ( 'NONE',  ( 0.5000000000000097700, 0.8660254037844329345, 0.000000000000000000 ) ) ;
#8353=CARTESIAN_POINT ( 'NONE',  ( 4.465502636338025688, -1.988169868018592856, -14.46874999795161720 ) ) ;
#8367=AXIS2_PLACEMENT_3D ( 'NONE', #2218, #19217, #17629 ) ;
#8369=CARTESIAN_POINT ( 'NONE',  ( -4.942249507334553371, 0.2590123213421660631, -10.34374999795161543 ) ) ;
#8374=CARTESIAN_POINT ( 'NONE',  ( -4.150607464521828938, -2.695436003842674566, -7.968749997951616315 ) ) ;
#8394=LINE ( 'NONE', #6869, #9996 ) ;
#8396=CARTESIAN_POINT ( 'NONE',  ( -2.849999999999989431, 4.936344801571308061, -7.312499995903225525 ) ) ;
#8407=CARTESIAN_POINT ( 'NONE',  ( -4.861323657744403448, 0.5109457054262118714, -13.84374999795161543 ) ) ;
#8441=ORIENTED_EDGE ( 'NONE', *, *, #13612, .F. ) ;
#8445=FACE_OUTER_BOUND ( 'NONE', #12306, .T. ) ;
#8472=CARTESIAN_POINT ( 'NONE',  ( -4.233219804643852946, 2.444050593750049405, -11.46874999795161543 ) ) ;
#8474=CARTESIAN_POINT ( 'NONE',  ( 2.647025296874957689, -4.584782303107616031, -7.078124996927420476 ) ) ;
#8482=CARTESIAN_POINT ( 'NONE',  ( -2.068159791354182708, 5.387740456496234565, -6.500000000000005329 ) ) ;
#8502=CARTESIAN_POINT ( 'NONE',  ( 4.781284448697187273, -1.016293382781444654, -10.84374999795161543 ) ) ;
#8504=CARTESIAN_POINT ( 'NONE',  ( 5.700000000000001066, 0.000000000000000000, -13.97977757194595760 ) ) ;
#8505=CARTESIAN_POINT ( 'NONE',  ( -3.499494075959816541, 3.499494075959816541, -9.343749997951615427 ) ) ;
#8509=CARTESIAN_POINT ( 'NONE',  ( 5.700000000000002842, 2.725425358843983450E-16, -10.64522241986047568 ) ) ;
#8519=CARTESIAN_POINT ( 'NONE',  ( 4.200000000000001066, 0.000000000000000000, 0.000000000000000000 ) ) ;
#8520=EDGE_LOOP ( 'NONE', ( #3112, #4541, #3044, #14985 ) ) ;
#8531=CARTESIAN_POINT ( 'NONE',  ( 0.5109457054261454800, -4.861323657744410554, -14.46874999795161720 ) ) ;
#8537=CARTESIAN_POINT ( 'NONE',  ( 4.080749450109621534, -4.080749450109678378, -9.812499995903223748 ) ) ;
#8540=CARTESIAN_POINT ( 'NONE',  ( 0.000000000000000000, 0.000000000000000000, -28.99999999999999645 ) ) ;
#8541=CARTESIAN_POINT ( 'NONE',  ( -4.080749450109677490, -4.080749450109622423, -13.50000000000000533 ) ) ;
#8564=CARTESIAN_POINT ( 'NONE',  ( -2.444050593750049849, -4.233219804643852946, -6.843749997951615427 ) ) ;
#8572=ORIENTED_EDGE ( 'NONE', *, *, #1660, .T. ) ;
#8592=CARTESIAN_POINT ( 'NONE',  ( 1.280903732194421663, -4.780397808154265960, -14.34374999795161365 ) ) ;
#8595=CARTESIAN_POINT ( 'NONE',  ( -4.648860486681953397, 1.510506337161861445, -7.843749997951614539 ) ) ;
#8609=CARTESIAN_POINT ( 'NONE',  ( 2.444050593750020095, 4.233219804643871598, -6.843749997951615427 ) ) ;
#8616=CARTESIAN_POINT ( 'NONE',  ( -5.142044285764751699, 2.620002426024544029, -8.812499995903225525 ) ) ;
#8622=LINE ( 'NONE', #4120, #847 ) ;
#8625=CARTESIAN_POINT ( 'NONE',  ( -2.246813503491864150, -4.409619785863891472, -13.34374999795161365 ) ) ;
#8630=B_SPLINE_CURVE_WITH_KNOTS ( 'NONE', 1,
 ( #15550, #15748 ),
 .UNSPECIFIED., .F., .F.,
 ( 2, 2 ),
 ( 0.000000000000000000, 1.000000000000000000 ),
 .UNSPECIFIED. ) ;
#8631=CARTESIAN_POINT ( 'NONE',  ( 0.9027913098498173694, -5.700000000000006395, -10.50000000000000533 ) ) ;
#8638=DIRECTION ( 'NONE',  ( 1.000000000000000000, 0.000000000000000000, 0.000000000000000000 ) ) ;
#8641=DIRECTION ( 'NONE',  ( 0.9945218953682738450, 0.1045284632676491549, 0.000000000000000000 ) ) ;
#8644=CARTESIAN_POINT ( 'NONE',  ( -0.7741991708319226895, -4.888101187499994893, -11.96874999795161365 ) ) ;
#8646=DIRECTION ( 'NONE',  ( -0.000000000000000000, -0.000000000000000000, 1.000000000000000000 ) ) ;
#8691=CARTESIAN_POINT ( 'NONE',  ( 4.781284448697187273, -1.016293382781444654, -10.46874999795161720 ) ) ;
#8704=B_SPLINE_CURVE_WITH_KNOTS ( 'NONE', 1,
 ( #17913, #2893 ),
 .UNSPECIFIED., .F., .F.,
 ( 2, 2 ),
 ( 0.000000000000000000, 1.000000000000000000 ),
 .UNSPECIFIED. ) ;
#8714=EDGE_CURVE ( 'NONE', #6321, #4362, #3384, .T. ) ;
#8717=CARTESIAN_POINT ( 'NONE',  ( 1.761396867937200073, 5.421022142882376826, -12.00000000000000533 ) ) ;
#8719=CARTESIAN_POINT ( 'NONE',  ( -1.988169868018624609, -4.465502636338009701, -9.468749997951615427 ) ) ;
#8721=ORIENTED_EDGE ( 'NONE', *, *, #2684, .T. ) ;
#8730=CARTESIAN_POINT ( 'NONE',  ( 4.861323657744406113, -0.5109457054261780096, -13.46874999795161543 ) ) ;
#8741=CARTESIAN_POINT ( 'NONE',  ( 0.7741991708318548548, -4.888101187500005551, -11.34374999795161543 ) ) ;
#8755=CARTESIAN_POINT ( 'NONE',  ( -5.294050593750000644, 0.000000000000000000, -7.078124996927420476 ) ) ;
#8760=CARTESIAN_POINT ( 'NONE',  ( -0.5109457054261112852, 4.861323657744413218, -14.84374999795161543 ) ) ;
#8764=CARTESIAN_POINT ( 'NONE',  ( 4.780397808154257078, -1.280903732194453859, -13.96874999795161365 ) ) ;
#8772=CARTESIAN_POINT ( 'NONE',  ( 3.143139765844623401, 4.840010801796481132, -9.500000000000005329 ) ) ;
#8788=CARTESIAN_POINT ( 'NONE',  ( -4.888101187500000222, 0.000000000000000000, -6.656249997951614539 ) ) ;
#8811=ORIENTED_EDGE ( 'NONE', *, *, #12380, .T. ) ;
#8818=CARTESIAN_POINT ( 'NONE',  ( 4.611396867937200383, 3.350375938067097881, -15.31249999590322552 ) ) ;
#8827=FACE_OUTER_BOUND ( 'NONE', #13812, .T. ) ;
#8828=CARTESIAN_POINT ( 'NONE',  ( 0.7741991708318548548, -4.888101187500005551, -11.34374999795161543 ) ) ;
#8844=CARTESIAN_POINT ( 'NONE',  ( -3.954556930911881096, -2.873153789725797935, -14.84374999795161543 ) ) ;
#8846=DIRECTION ( 'NONE',  ( 1.000000000000000000, 0.000000000000000000, 0.000000000000000000 ) ) ;
#8860=( BOUNDED_SURFACE ( )  B_SPLINE_SURFACE ( 1, 2, ( 
 ( #16184, #6551, #5364, #8374, #10083, #16084, #17481, #12781, #2455, #3669, #12683, #9791, #11570, #5458, #11477, #18879, #5067 ),
 ( #14177, #17577, #18774, #8272, #9984, #9690, #14380, #3770, #14490, #6852, #15885, #3865, #11180, #480, #15783, #678, #12880 ) ),
 .UNSPECIFIED., .F., .F., .F. ) 
 B_SPLINE_SURFACE_WITH_KNOTS ( ( 2, 2 ),
 ( 3, 2, 2, 2, 2, 2, 2, 2, 3 ),
 ( 0.000000000000000000, 1.000000000000000000 ),
 ( 0.000000000000000000, 0.05000000000000000278, 0.1000000000000000056, 0.1499999999999999944, 0.2000000000000000111, 0.2500000000000000000, 0.2999999999999999889, 0.3499999999999999778, 0.4000000000000000222 ),
 .UNSPECIFIED. ) 
 GEOMETRIC_REPRESENTATION_ITEM ( )  RATIONAL_B_SPLINE_SURFACE ( (
 ( 1.000000000000000000, 0.9876883405951377704, 1.000000000000000000, 0.9876883405951377704, 1.000000000000000000, 0.9876883405951377704, 1.000000000000000000, 0.9876883405951377704, 1.000000000000000000, 0.9876883405951377704, 1.000000000000000000, 0.9876883405951377704, 1.000000000000000000, 0.9876883405951377704, 1.000000000000000000, 0.9876883405951377704, 1.000000000000000000),
 ( 1.000000000000000000, 0.9876883405951377704, 1.000000000000000000, 0.9876883405951377704, 1.000000000000000000, 0.9876883405951377704, 1.000000000000000000, 0.9876883405951377704, 1.000000000000000000, 0.9876883405951377704, 1.000000000000000000, 0.9876883405951377704, 1.000000000000000000, 0.9876883405951377704, 1.000000000000000000, 0.9876883405951377704, 1.000000000000000000) ) ) 
 REPRESENTATION_ITEM ( '' )  SURFACE ( )  );
#8881=CARTESIAN_POINT ( 'NONE',  ( -0.9027913098498963063, -5.699999999999994849, -12.81249999590322552 ) ) ;
#8890=CARTESIAN_POINT ( 'NONE',  ( 5.700000000000001954, 0.000000000000000000, 0.000000000000000000 ) ) ;
#8893=CARTESIAN_POINT ( 'NONE',  ( -4.235925505221191933, -3.814044456245443193, -8.312499995903225525 ) ) ;
#8897=CARTESIAN_POINT ( 'NONE',  ( -4.780397808154273953, -1.280903732194386579, -8.968749997951613651 ) ) ;
#8919=VERTEX_POINT ( 'NONE', #5754 ) ;
#8925=CARTESIAN_POINT ( 'NONE',  ( -2.873153789725852558, -3.954556930911842016, -13.84374999795161543 ) ) ;
#8928=CARTESIAN_POINT ( 'NONE',  ( 4.233219804643887585, 2.444050593749990785, -11.84374999795161365 ) ) ;
#8931=VERTEX_POINT ( 'NONE', #16281 ) ;
#8941=CARTESIAN_POINT ( 'NONE',  ( -1.510506337161893642, -4.648860486681943627, -12.84374999795161543 ) ) ;
#8944=ORIENTED_EDGE ( 'NONE', *, *, #17472, .T. ) ;
#8950=EDGE_CURVE ( 'NONE', #10504, #12259, #11711, .T. ) ;
#8957=CARTESIAN_POINT ( 'NONE',  ( 2.695436003842732298, 4.150607464521791634, -9.968749997951615427 ) ) ;
#8968=ORIENTED_EDGE ( 'NONE', *, *, #15427, .T. ) ;
#8975=( BOUNDED_CURVE ( )  B_SPLINE_CURVE ( 2, ( #8396, #5290, #11198, #14298, #1160, #14402, #3689, #6573, #7234, #18796, #8192, #3592, #6871, #18997, #8089 ),
 .UNSPECIFIED., .F., .F. ) 
 B_SPLINE_CURVE_WITH_KNOTS ( ( 3, 2, 2, 2, 2, 2, 2, 3 ),
 ( 0.000000000000000000, 0.05000000000000000971, 0.1000000000000000194, 0.1499999999999999944, 0.2000000000000000389, 0.2500000000000000000, 0.2999999999999999889, 0.3333180920165872418 ),
 .UNSPECIFIED. ) 
 CURVE ( )  GEOMETRIC_REPRESENTATION_ITEM ( )  RATIONAL_B_SPLINE_CURVE ( ( 1.000000000000000000, 0.9876883405951377704, 1.000000000000000000, 0.9876883405951377704, 1.000000000000000000, 0.9876883405951377704, 1.000000000000000000, 0.9876883405951377704, 1.000000000000000000, 0.9876883405951377704, 1.000000000000000000, 0.9876883405951377704, 1.000000000000000000, 0.9917959799814383137, 0.9945256517182510247 ) ) 
 REPRESENTATION_ITEM ( '' )  );
#8978=CARTESIAN_POINT ( 'NONE',  ( -0.5109457054261112852, 4.861323657744413218, -14.46874999795161720 ) ) ;
#8990=CARTESIAN_POINT ( 'NONE',  ( 4.620319390059819398, -1.773574444220757496, -10.96874999795161720 ) ) ;
#8996=CARTESIAN_POINT ( 'NONE',  ( -4.861323657744413218, -0.5109457054261099529, -9.468749997951615427 ) ) ;
#9005=CARTESIAN_POINT ( 'NONE',  ( 0.000000000000000000, 0.000000000000000000, 0.000000000000000000 ) ) ;
#9017=ORIENTED_EDGE ( 'NONE', *, *, #16236, .T. ) ;
#9024=CARTESIAN_POINT ( 'NONE',  ( -2.993098736590125853E-16, 4.888101187500000222, -11.84374999795161365 ) ) ;
#9025=CARTESIAN_POINT ( 'NONE',  ( -0.7741991708319226895, -4.888101187499994893, -12.34374999795161543 ) ) ;
#9037=AXIS2_PLACEMENT_3D ( 'NONE', #15351, #4831, #18346 ) ;
#9060=CARTESIAN_POINT ( 'NONE',  ( 4.620319390059829168, 1.773574444220725299, -11.96874999795161365 ) ) ;
#9061=VERTEX_POINT ( 'NONE', #18181 ) ;
#9065=ORIENTED_EDGE ( 'NONE', *, *, #10561, .F. ) ;
#9095=CARTESIAN_POINT ( 'NONE',  ( 3.499494075959815653, 3.499494075959816541, -14.34374999795161365 ) ) ;
#9117=EDGE_CURVE ( 'NONE', #13431, #13685, #6773, .T. ) ;
#9121=CARTESIAN_POINT ( 'NONE',  ( -1.280903732194487166, -4.780397808154247308, -9.343749997951615427 ) ) ;
#9126=CARTESIAN_POINT ( 'NONE',  ( 2.873153789725825025, 3.954556930911862000, -13.84374999795161543 ) ) ;
#9142=DIRECTION ( 'NONE',  ( -0.4330127018922180770, 0.7500000000000021094, 0.4999999999999979461 ) ) ;
#9147=EDGE_CURVE ( 'NONE', #5524, #10504, #6914, .T. ) ;
#9157=CARTESIAN_POINT ( 'NONE',  ( -4.936344801571268093, 2.850000000000057820, -12.31249999590322552 ) ) ;
#9159=CARTESIAN_POINT ( 'NONE',  ( 0.000000000000000000, 0.000000000000000000, -6.000000000000005329 ) ) ;
#9160=ORIENTED_EDGE ( 'NONE', *, *, #7008, .F. ) ;
#9161=CARTESIAN_POINT ( 'NONE',  ( 4.465502636338025688, -1.988169868018592856, -14.46874999795161720 ) ) ;
#9164=EDGE_CURVE ( 'NONE', #2645, #4579, #4246, .T. ) ;
#9168=CARTESIAN_POINT ( 'NONE',  ( 1.988169868018593300, 4.465502636338024800, -9.843749997951615427 ) ) ;
#9177=AXIS2_PLACEMENT_3D ( 'NONE', #431, #3429, #16946 ) ;
#9181=EDGE_LOOP ( 'NONE', ( #12320, #8572, #7069, #3183 ) ) ;
#9199=FACE_OUTER_BOUND ( 'NONE', #5449, .T. ) ;
#9210=CARTESIAN_POINT ( 'NONE',  ( 2.695436003842704764, -4.150607464521811174, -13.34374999795161365 ) ) ;
#9226=EDGE_CURVE ( 'NONE', #5242, #13431, #19443, .T. ) ;
#9227=ADVANCED_FACE ( 'NONE', ( #13440, #13156 ), #19344, .F. ) ;
#9241=CARTESIAN_POINT ( 'NONE',  ( -5.700000000000001066, 1.090170143537592985E-15, -9.332722423957234170 ) ) ;
#9247=VERTEX_POINT ( 'NONE', #17663 ) ;
#9255=EDGE_LOOP ( 'NONE', ( #19716, #8271, #10325, #4058, #5899 ) ) ;
#9257=CARTESIAN_POINT ( 'NONE',  ( -5.700000000000001066, 1.090170143537592985E-15, -10.64522241986045259 ) ) ;
#9284=ORIENTED_EDGE ( 'NONE', *, *, #4503, .F. ) ;
#9289=CARTESIAN_POINT ( 'NONE',  ( -3.499494075959816541, 3.499494075959816541, -8.968749997951611874 ) ) ;
#9324=CARTESIAN_POINT ( 'NONE',  ( 0.7741991708318884946, 4.888101187500000222, -11.96874999795161365 ) ) ;
#9336=B_SPLINE_CURVE_WITH_KNOTS ( 'NONE', 1,
 ( #15844, #12647 ),
 .UNSPECIFIED., .F., .F.,
 ( 2, 2 ),
 ( 0.000000000000000000, 1.000000000000000000 ),
 .UNSPECIFIED. ) ;
#9354=AXIS2_PLACEMENT_3D ( 'NONE', #17072, #16783, #19672 ) ;
#9363=AXIS2_PLACEMENT_3D ( 'NONE', #11762, #3048, #19754 ) ;
#9365=ORIENTED_EDGE ( 'NONE', *, *, #15682, .T. ) ;
#9373=ADVANCED_FACE ( 'NONE', ( #7421 ), #13546, .T. ) ;
#9378=CARTESIAN_POINT ( 'NONE',  ( 4.200000000000001954, 0.000000000000000000, -6.000000000000005329 ) ) ;
#9393=CARTESIAN_POINT ( 'NONE',  ( -2.444050593750049849, -4.233219804643852946, -6.843749997951615427 ) ) ;
#9406=CARTESIAN_POINT ( 'NONE',  ( -0.9027913098498961952, -5.699999999999994849, -11.50000000000000355 ) ) ;
#9428=VECTOR ( 'NONE', #6985, 1000.000000000000000 ) ;
#9441=FACE_OUTER_BOUND ( 'NONE', #19138, .T. ) ;
#9443=CARTESIAN_POINT ( 'NONE',  ( -5.700000000000001066, -0.2987243419133009947, -9.165444847914514526 ) ) ;
#9462=ORIENTED_EDGE ( 'NONE', *, *, #14281, .F. ) ;
#9466=ORIENTED_EDGE ( 'NONE', *, *, #11919, .F. ) ;
#9469=B_SPLINE_CURVE_WITH_KNOTS ( 'NONE', 1,
 ( #5309, #10215 ),
 .UNSPECIFIED., .F., .F.,
 ( 2, 2 ),
 ( 0.000000000000000000, 1.000000000000000000 ),
 .UNSPECIFIED. ) ;
#9471=EDGE_CURVE ( 'NONE', #12976, #4769, #5202, .T. ) ;
#9474=AXIS2_PLACEMENT_3D ( 'NONE', #12421, #4911, #8106 ) ;
#9489=ADVANCED_BREP_SHAPE_REPRESENTATION ( '', ( #16364, #16724 ), #15776 ) ;
#9493=CARTESIAN_POINT ( 'NONE',  ( -4.936344801571268093, 2.850000000000057820, -12.31249999590322552 ) ) ;
#9494=ORIENTED_EDGE ( 'NONE', *, *, #6590, .F. ) ;
#9495=DIRECTION ( 'NONE',  ( 0.000000000000000000, 0.000000000000000000, -1.000000000000000000 ) ) ;
#9504=CARTESIAN_POINT ( 'NONE',  ( 2.620002426024508502, -5.142044285764769462, -9.500000000000003553 ) ) ;
#9505=VERTEX_POINT ( 'NONE', #11320 ) ;
#9507=( LENGTH_UNIT ( ) NAMED_UNIT ( * ) SI_UNIT ( .MILLI., .METRE. ) );
#9508=CARTESIAN_POINT ( 'NONE',  ( -3.954556930911881096, -2.873153789725797935, -14.46874999795161720 ) ) ;
#9512=VECTOR ( 'NONE', #16135, 1000.000000000000000 ) ;
#9515=CIRCLE ( 'NONE', #6936, 5.700000000000002842 ) ;
#9519=CARTESIAN_POINT ( 'NONE',  ( -4.200000000000001066, 5.143516556418885886E-16, 0.000000000000000000 ) ) ;
#9520=CARTESIAN_POINT ( 'NONE',  ( 0.7741991708318884946, 4.888101187500000222, -12.34374999795161543 ) ) ;
#9535=CARTESIAN_POINT ( 'NONE',  ( 5.700000000000001954, 0.000000000000000000, 0.000000000000000000 ) ) ;
#9542=CARTESIAN_POINT ( 'NONE',  ( 0.5109457054261454800, -4.861323657744410554, -14.84374999795161543 ) ) ;
#9551=CARTESIAN_POINT ( 'NONE',  ( 0.2590123213420630899, -4.942249507334558700, -7.968749997951616315 ) ) ;
#9574=CARTESIAN_POINT ( 'NONE',  ( -4.936344801571327601, -2.849999999999954792, -11.00000000000000711 ) ) ;
#9586=CARTESIAN_POINT ( 'NONE',  ( 1.510506337161861223, 4.648860486681953397, -12.46874999795161543 ) ) ;
#9605=CARTESIAN_POINT ( 'NONE',  ( 5.207209108562820710, -2.318398865532075526, 0.000000000000000000 ) ) ;
#9611=LINE ( 'NONE', #3404, #7618 ) ;
#9622=EDGE_CURVE ( 'NONE', #17426, #5986, #12954, .T. ) ;
#9631=CARTESIAN_POINT ( 'NONE',  ( -2.318398865532001363, 5.207209108562852684, -14.31249999590322552 ) ) ;
#9634=DIRECTION ( 'NONE',  ( 1.000000000000000000, 0.000000000000000000, 0.000000000000000000 ) ) ;
#9642=FACE_OUTER_BOUND ( 'NONE', #12965, .T. ) ;
#9650=CARTESIAN_POINT ( 'NONE',  ( 3.954556930911861112, 2.873153789725825913, -14.46874999795161720 ) ) ;
#9658=FACE_OUTER_BOUND ( 'NONE', #3022, .T. ) ;
#9672=EDGE_CURVE ( 'NONE', #8919, #2645, #13897, .T. ) ;
#9673=CARTESIAN_POINT ( 'NONE',  ( -3.114526743279308896, -3.846120219227900705, -7.343749997951615427 ) ) ;
#9677=EDGE_CURVE ( 'NONE', #12952, #1346, #7629, .T. ) ;
#9690=CARTESIAN_POINT ( 'NONE',  ( -5.574407415329178939, -1.493657965219446382, -8.500000000000007105 ) ) ;
#9695=CARTESIAN_POINT ( 'NONE',  ( -3.350375938067097437, 4.611396867937201272, -9.000000000000005329 ) ) ;
#9704=DIRECTION ( 'NONE',  ( 1.000000000000000000, 0.000000000000000000, 0.000000000000000000 ) ) ;
#9708=CARTESIAN_POINT ( 'NONE',  ( -2.620002426024580000, -5.142044285764733935, -12.50000000000000533 ) ) ;
#9717=CARTESIAN_POINT ( 'NONE',  ( 2.444050593750020095, 4.233219804643871598, -6.843749997951615427 ) ) ;
#9742=CARTESIAN_POINT ( 'NONE',  ( 3.143139765844590983, -4.840010801796506001, -13.81249999590322730 ) ) ;
#9748=CARTESIAN_POINT ( 'NONE',  ( 3.114526743279282694, 3.846120219227923798, -7.343749997951615427 ) ) ;
#9754=( BOUNDED_CURVE ( )  B_SPLINE_CURVE ( 2, ( #1996, #17111, #12414, #3402, #7695, #8095, #6192, #6287, #18507, #1708, #4997 ),
 .UNSPECIFIED., .F., .F. ) 
 B_SPLINE_CURVE_WITH_KNOTS ( ( 3, 2, 2, 2, 2, 3 ),
 ( 0.1666819079834116757, 0.2000000000000000111, 0.2500000000000000000, 0.2999999999999999889, 0.3499999999999999778, 0.4000000000000000222 ),
 .UNSPECIFIED. ) 
 CURVE ( )  GEOMETRIC_REPRESENTATION_ITEM ( )  RATIONAL_B_SPLINE_CURVE ( ( 0.9945256517182512468, 0.9917959799814380917, 1.000000000000000000, 0.9876883405951377704, 1.000000000000000000, 0.9876883405951377704, 1.000000000000000000, 0.9876883405951377704, 1.000000000000000000, 0.9876883405951377704, 1.000000000000000000 ) ) 
 REPRESENTATION_ITEM ( '' )  );
#9758=CARTESIAN_POINT ( 'NONE',  ( -4.942249507334558700, -0.2590123213420630899, -12.96874999795161543 ) ) ;
#9770=B_SPLINE_CURVE_WITH_KNOTS ( 'NONE', 1,
 ( #11719, #5700 ),
 .UNSPECIFIED., .F., .F.,
 ( 2, 2 ),
 ( 0.000000000000000000, 1.000000000000000000 ),
 .UNSPECIFIED. ) ;
#9771=ORIENTED_EDGE ( 'NONE', *, *, #15518, .F. ) ;
#9779=CIRCLE ( 'NONE', #12639, 9.000000000000001776 ) ;
#9791=CARTESIAN_POINT ( 'NONE',  ( -3.846120219227901593, 3.114526743279308896, -11.96874999795161365 ) ) ;
#9811=DIRECTION ( 'NONE',  ( -0.8660254037844398178, 6.047423072554923456E-15, 0.4999999999999979461 ) ) ;
#9814=CARTESIAN_POINT ( 'NONE',  ( 4.840010801796506890, 3.143139765844590983, -8.812499995903225525 ) ) ;
#9820=CARTESIAN_POINT ( 'NONE',  ( -5.700000000000001066, 0.000000000000000000, -7.312499995903225525 ) ) ;
#9826=CARTESIAN_POINT ( 'NONE',  ( -4.611396867937226141, -3.350375938067064574, 0.000000000000000000 ) ) ;
#9833=DIRECTION ( 'NONE',  ( 0.000000000000000000, 0.000000000000000000, 1.000000000000000000 ) ) ;
#9845=CARTESIAN_POINT ( 'NONE',  ( 1.761396867937200073, 5.421022142882376826, -13.31249999590322730 ) ) ;
#9848=CARTESIAN_POINT ( 'NONE',  ( 4.150607464521812062, 2.695436003842704764, -8.343749997951611874 ) ) ;
#9859=EDGE_CURVE ( 'NONE', #5986, #17426, #9779, .T. ) ;
#9866=VECTOR ( 'NONE', #9811, 1000.000000000000000 ) ;
#9885=CARTESIAN_POINT ( 'NONE',  ( -4.150607464521828938, -2.695436003842674566, -7.968749997951616315 ) ) ;
#9888=CARTESIAN_POINT ( 'NONE',  ( 3.846120219227944670, 3.114526743279255161, -10.96874999795161720 ) ) ;
#9918=CARTESIAN_POINT ( 'NONE',  ( -4.781284448697201483, -1.016293382781378485, -12.84374999795161543 ) ) ;
#9930=CARTESIAN_POINT ( 'NONE',  ( -5.700000000000001954, 6.980486755139915080E-16, 0.000000000000000000 ) ) ;
#9950=VECTOR ( 'NONE', #5938, 1000.000000000000000 ) ;
#9953=CARTESIAN_POINT ( 'NONE',  ( -0.9027913098498961952, -5.699999999999994849, -12.81249999590322552 ) ) ;
#9955=EDGE_LOOP ( 'NONE', ( #16460, #7523, #1343, #4063 ) ) ;
#9957=CARTESIAN_POINT ( 'NONE',  ( -0.7741991708319226895, -4.888101187499994893, -11.96874999795161365 ) ) ;
#9958=CARTESIAN_POINT ( 'NONE',  ( 5.700000000000002842, 2.725425358843983450E-16, -10.64522241986047568 ) ) ;
#9980=CARTESIAN_POINT ( 'NONE',  ( 4.620319390059829168, 1.773574444220725299, -11.96874999795161365 ) ) ;
#9984=CARTESIAN_POINT ( 'NONE',  ( -5.207209108562852684, -2.318398865532001363, -8.000000000000005329 ) ) ;
#9996=VECTOR ( 'NONE', #19282, 1000.000000000000000 ) ;
#10011=CARTESIAN_POINT ( 'NONE',  ( 3.143139765844590983, -4.840010801796506890, -13.81249999590322552 ) ) ;
#10012=VECTOR ( 'NONE', #8269, 1000.000000000000000 ) ;
#10014=PLANE ( 'NONE',  #5497 ) ;
#10016=CARTESIAN_POINT ( 'NONE',  ( -4.620319390059842490, -1.773574444220693325, -12.34374999795161543 ) ) ;
#10049=DIRECTION ( 'NONE',  ( -0.000000000000000000, -0.000000000000000000, 1.000000000000000000 ) ) ;
#10057=ADVANCED_FACE ( 'NONE', ( #19152 ), #3848, .T. ) ;
#10078=CARTESIAN_POINT ( 'NONE',  ( -4.620319390059805187, 1.773574444220790136, -11.34374999795161543 ) ) ;
#10083=CARTESIAN_POINT ( 'NONE',  ( -4.465502636338051445, -1.988169868018530462, -8.468749997951615427 ) ) ;
#10091=ORIENTED_EDGE ( 'NONE', *, *, #6025, .T. ) ;
#10104=CARTESIAN_POINT ( 'NONE',  ( 5.763142191869155440, -0.3020334839682879413, -10.81249999590322375 ) ) ;
#10106=CARTESIAN_POINT ( 'NONE',  ( -2.620002426024544473, 5.142044285764749922, -10.81249999590322375 ) ) ;
#10114=EDGE_CURVE ( 'NONE', #1346, #11278, #5799, .T. ) ;
#10129=CARTESIAN_POINT ( 'NONE',  ( 2.620002426024544029, 5.142044285764751699, -13.81249999590322730 ) ) ;
#10140=CARTESIAN_POINT ( 'NONE',  ( -4.080749450109677490, -4.080749450109621534, -14.81249999590322552 ) ) ;
#10180=EDGE_LOOP ( 'NONE', ( #2210, #16284, #9365, #13956 ) ) ;
#10190=PRODUCT_DEFINITION_SHAPE ( 'NONE', 'NONE',  #7325 ) ;
#10195=ORIENTED_EDGE ( 'NONE', *, *, #15579, .F. ) ;
#10198=UNCERTAINTY_MEASURE_WITH_UNIT (LENGTH_MEASURE( 1.000000000000000082E-05 ), #7311, 'distance_accuracy_value', 'NONE');
#10203=CARTESIAN_POINT ( 'NONE',  ( 4.611396867937200383, 3.350375938067097881, -15.31249999590322552 ) ) ;
#10215=CARTESIAN_POINT ( 'NONE',  ( -4.611396867937224364, -3.350375938067065906, -15.31249999590322552 ) ) ;
#10231=ORIENTED_EDGE ( 'NONE', *, *, #17245, .F. ) ;
#10232=CARTESIAN_POINT ( 'NONE',  ( -4.465502636338010589, 1.988169868018623720, -14.84374999795161543 ) ) ;
#10236=EDGE_CURVE ( 'NONE', #13685, #19526, #4123, .T. ) ;
#10238=CARTESIAN_POINT ( 'NONE',  ( 4.409619785863891472, -2.246813503491864150, -8.343749997951611874 ) ) ;
#10241=CARTESIAN_POINT ( 'NONE',  ( -1.016293382781411125, 4.781284448697194378, -7.843749997951614539 ) ) ;
#10250=ORIENTED_EDGE ( 'NONE', *, *, #12772, .F. ) ;
#10268=( BOUNDED_SURFACE ( )  B_SPLINE_SURFACE ( 1, 2, ( 
 ( #231, #6314, #17042, #14034, #328, #4253, #16657, #2740, #5841, #12258, #3145, #6137, #15263, #13553, #1350, #4449, #18063 ),
 ( #1550, #7534, #13351, #18258, #7639, #19547, #15057, #10659, #13446, #4545, #10365, #7430, #19656, #2842, #13654, #19749, #4646 ) ),
 .UNSPECIFIED., .F., .F., .F. ) 
 B_SPLINE_SURFACE_WITH_KNOTS ( ( 2, 2 ),
 ( 3, 2, 2, 2, 2, 2, 2, 2, 3 ),
 ( 0.000000000000000000, 1.000000000000000000 ),
 ( 0.000000000000000000, 0.05000000000000000278, 0.1000000000000000056, 0.1499999999999999944, 0.2000000000000000111, 0.2500000000000000000, 0.2999999999999999889, 0.3499999999999999778, 0.4000000000000000222 ),
 .UNSPECIFIED. ) 
 GEOMETRIC_REPRESENTATION_ITEM ( )  RATIONAL_B_SPLINE_SURFACE ( (
 ( 1.000000000000000000, 0.9876883405951377704, 1.000000000000000000, 0.9876883405951377704, 1.000000000000000000, 0.9876883405951377704, 1.000000000000000000, 0.9876883405951377704, 1.000000000000000000, 0.9876883405951377704, 1.000000000000000000, 0.9876883405951377704, 1.000000000000000000, 0.9876883405951377704, 1.000000000000000000, 0.9876883405951377704, 1.000000000000000000),
 ( 1.000000000000000000, 0.9876883405951377704, 1.000000000000000000, 0.9876883405951377704, 1.000000000000000000, 0.9876883405951377704, 1.000000000000000000, 0.9876883405951377704, 1.000000000000000000, 0.9876883405951377704, 1.000000000000000000, 0.9876883405951377704, 1.000000000000000000, 0.9876883405951377704, 1.000000000000000000, 0.9876883405951377704, 1.000000000000000000) ) ) 
 REPRESENTATION_ITEM ( '' )  SURFACE ( )  );
#10277=CARTESIAN_POINT ( 'NONE',  ( -2.849999999999989431, 4.936344801571308061, -7.312499995903225525 ) ) ;
#10317=ADVANCED_FACE ( 'NONE', ( #16850 ), #10268, .T. ) ;
#10320=CARTESIAN_POINT ( 'NONE',  ( 4.620319390059819398, -1.773574444220757496, -11.34374999795161543 ) ) ;
#10324=LINE ( 'NONE', #19706, #2156 ) ;
#10325=ORIENTED_EDGE ( 'NONE', *, *, #15785, .T. ) ;
#10333=ORIENTED_EDGE ( 'NONE', *, *, #11485, .T. ) ;
#10341=ORIENTED_EDGE ( 'NONE', *, *, #11919, .T. ) ;
#10343=CARTESIAN_POINT ( 'NONE',  ( -0.2590123213420971182, 4.942249507334556924, -8.343749997951611874 ) ) ;
#10365=CARTESIAN_POINT ( 'NONE',  ( 4.936344801571289409, -2.850000000000023626, -11.00000000000000711 ) ) ;
#10372=CARTESIAN_POINT ( 'NONE',  ( -4.620319390059841602, -1.773574444220693325, -11.96874999795161365 ) ) ;
#10397=VECTOR ( 'NONE', #1692, 1000.000000000000114 ) ;
#10424=AXIS2_PLACEMENT_3D ( 'NONE', #13138, #16242, #8341 ) ;
#10425=CARTESIAN_POINT ( 'NONE',  ( 4.861323657744407001, -0.5109457054261775655, -13.84374999795161543 ) ) ;
#10427=CARTESIAN_POINT ( 'NONE',  ( -4.942249507334558700, -0.2590123213420631454, -13.34374999795161365 ) ) ;
#10433=CARTESIAN_POINT ( 'NONE',  ( -2.246813503491833508, 4.409619785863906571, -10.34374999795161543 ) ) ;
#10437=CARTESIAN_POINT ( 'NONE',  ( 4.465502636338025688, -1.988169868018592856, -14.46874999795161720 ) ) ;
#10443=DIRECTION ( 'NONE',  ( 6.982962677686267499E-15, 1.000000000000000000, -0.000000000000000000 ) ) ;
#10468=CARTESIAN_POINT ( 'NONE',  ( 2.068159791354145849, -5.387740456496247887, -6.500000000000005329 ) ) ;
#10475=ORIENTED_EDGE ( 'NONE', *, *, #216, .T. ) ;
#10487=CARTESIAN_POINT ( 'NONE',  ( 5.700000000000001066, -3.980288726281172656E-14, -7.312499995903225525 ) ) ;
#10489=ADVANCED_FACE ( 'NONE', ( #4130 ), #2139, .F. ) ;
#10500=ORIENTED_EDGE ( 'NONE', *, *, #13305, .F. ) ;
#10502=( BOUNDED_CURVE ( )  B_SPLINE_CURVE ( 2, ( #13928, #221, #7509, #19727, #10633, #16738, #3017, #15237, #6113, #7910, #8009, #12529, #6500, #14225, #6598, #8315, #14325 ),
 .UNSPECIFIED., .F., .F. ) 
 B_SPLINE_CURVE_WITH_KNOTS ( ( 3, 2, 2, 2, 2, 2, 2, 2, 3 ),
 ( 0.000000000000000000, 0.05000000000000000971, 0.1000000000000000194, 0.1499999999999999944, 0.2000000000000000389, 0.2500000000000000000, 0.2999999999999999889, 0.3499999999999999223, 0.4000000000000000777 ),
 .UNSPECIFIED. ) 
 CURVE ( )  GEOMETRIC_REPRESENTATION_ITEM ( )  RATIONAL_B_SPLINE_CURVE ( ( 1.000000000000000000, 0.9876883405951377704, 1.000000000000000000, 0.9876883405951377704, 1.000000000000000000, 0.9876883405951377704, 1.000000000000000000, 0.9876883405951377704, 1.000000000000000000, 0.9876883405951377704, 1.000000000000000000, 0.9876883405951377704, 1.000000000000000000, 0.9876883405951377704, 1.000000000000000000, 0.9876883405951377704, 1.000000000000000000 ) ) 
 REPRESENTATION_ITEM ( '' )  );
#10503=CARTESIAN_POINT ( 'NONE',  ( -3.632567103900569361, -3.270778111535287191, -7.468749997951615427 ) ) ;
#10504=VERTEX_POINT ( 'NONE', #2424 ) ;
#10519=EDGE_CURVE ( 'NONE', #488, #4769, #1557, .T. ) ;
#10524=CARTESIAN_POINT ( 'NONE',  ( 0.2590123213420631454, -4.942249507334558700, -7.968749997951616315 ) ) ;
#10527=EDGE_CURVE ( 'NONE', #15763, #2089, #4761, .T. ) ;
#10528=CARTESIAN_POINT ( 'NONE',  ( -2.246813503491833508, 4.409619785863906571, -9.968749997951617203 ) ) ;
#10530=ORIENTED_EDGE ( 'NONE', *, *, #13662, .F. ) ;
#10561=EDGE_CURVE ( 'NONE', #14057, #17046, #5714, .T. ) ;
#10571=CARTESIAN_POINT ( 'NONE',  ( 4.620319390059829168, 1.773574444220725743, -12.34374999795161543 ) ) ;
#10629=CARTESIAN_POINT ( 'NONE',  ( 3.954556930911842016, -2.873153789725853002, -8.843749997951615427 ) ) ;
#10631=CARTESIAN_POINT ( 'NONE',  ( 3.270778111535338262, 3.632567103900523620, -10.46874999795161720 ) ) ;
#10633=CARTESIAN_POINT ( 'NONE',  ( -3.954556930911862000, 2.873153789725825469, -8.468749997951615427 ) ) ;
#10642=CARTESIAN_POINT ( 'NONE',  ( 5.294050593750000644, -3.696815770993907903E-14, -6.234374998975811266 ) ) ;
#10653=ORIENTED_EDGE ( 'NONE', *, *, #16064, .T. ) ;
#10659=CARTESIAN_POINT ( 'NONE',  ( 5.763142191869155440, -0.3020334839682879413, -9.500000000000003553 ) ) ;
#10670=MECHANICAL_DESIGN_GEOMETRIC_PRESENTATION_REPRESENTATION('',(#17051),#16419);
#10671=CARTESIAN_POINT ( 'NONE',  ( -1.185096637661215535, 5.575441324182696334, -8.312499995903225525 ) ) ;
#10679=EDGE_CURVE ( 'NONE', #9247, #15763, #3419, .T. ) ;
#10694=CARTESIAN_POINT ( 'NONE',  ( -0.7741991708318890497, 4.888101187500000222, -11.34374999795161543 ) ) ;
#10717=LINE ( 'NONE', #9519, #12524 ) ;
#10723=AXIS2_PLACEMENT_3D ( 'NONE', #17463, #19056, #7025 ) ;
#10726=LINE ( 'NONE', #1423, #3569 ) ;
#10728=ORIENTED_EDGE ( 'NONE', *, *, #6593, .F. ) ;
#10731=ORIENTED_EDGE ( 'NONE', *, *, #16768, .T. ) ;
#10745=FACE_OUTER_BOUND ( 'NONE', #7185, .T. ) ;
#10788=CARTESIAN_POINT ( 'NONE',  ( -4.942249507334553371, 0.2590123213421660631, -10.34374999795161543 ) ) ;
#10816=CARTESIAN_POINT ( 'NONE',  ( 4.233219804643887585, 2.444050593749991229, -11.84374999795161365 ) ) ;
#10829=ORIENTED_EDGE ( 'NONE', *, *, #3310, .F. ) ;
#10832=VECTOR ( 'NONE', #17210, 1000.000000000000114 ) ;
#10836=CARTESIAN_POINT ( 'NONE',  ( 2.444050593749960587, -4.233219804643904460, -6.843749997951615427 ) ) ;
#10837=CARTESIAN_POINT ( 'NONE',  ( -4.840010801796527318, -3.143139765844555900, -7.500000000000005329 ) ) ;
#10849=DIRECTION ( 'NONE',  ( -0.000000000000000000, -0.000000000000000000, 1.000000000000000000 ) ) ;
#10858=CARTESIAN_POINT ( 'NONE',  ( -2.318398865532109721, -5.207209108562803834, -9.000000000000005329 ) ) ;
#10884=CARTESIAN_POINT ( 'NONE',  ( -5.575441324182703440, -1.185096637661177343, -13.31249999590322730 ) ) ;
#10888=CARTESIAN_POINT ( 'NONE',  ( -4.888101187500000222, 0.000000000000000000, -6.468749997951615427 ) ) ;
#10908=EDGE_CURVE ( 'NONE', #12853, #16351, #15583, .T. ) ;
#10923=CARTESIAN_POINT ( 'NONE',  ( 5.700000000000001066, -3.980288726281172656E-14, -7.312499995903225525 ) ) ;
#10927=ADVANCED_FACE ( 'NONE', ( #16609 ), #12109, .T. ) ;
#10933=ORIENTED_EDGE ( 'NONE', *, *, #17138, .T. ) ;
#10939=CARTESIAN_POINT ( 'NONE',  ( 3.270778111535314281, -3.632567103900546712, -12.46874999795161543 ) ) ;
#10959=CARTESIAN_POINT ( 'NONE',  ( 0.3020334839682081163, -5.763142191869158992, -7.500000000000005329 ) ) ;
#10963=ORIENTED_EDGE ( 'NONE', *, *, #51, .F. ) ;
#10972=CARTESIAN_POINT ( 'NONE',  ( -5.700000000000001066, -0.5990941410143296730, -12.33180101230370518 ) ) ;
#10982=LINE ( 'NONE', #7965, #7339 ) ;
#10985=CARTESIAN_POINT ( 'NONE',  ( -2.873153789725825469, 3.954556930911862000, -9.468749997951615427 ) ) ;
#10997=CARTESIAN_POINT ( 'NONE',  ( 4.888101187500000222, -3.413342815706642518E-14, -6.468749997951615427 ) ) ;
#11009=CARTESIAN_POINT ( 'NONE',  ( -2.993098736590125853E-16, 4.888101187500000222, -11.84374999795161365 ) ) ;
#11022=( BOUNDED_CURVE ( )  B_SPLINE_CURVE ( 2, ( #6684, #3203, #15418, #14013, #1714, #7802, #18512, #306, #12516, #18609, #11009, #9520, #15615, #14107, #17701, #3894, #707 ),
 .UNSPECIFIED., .F., .F. ) 
 B_SPLINE_CURVE_WITH_KNOTS ( ( 3, 2, 2, 2, 2, 2, 2, 2, 3 ),
 ( 0.000000000000000000, 0.05000000000000000971, 0.1000000000000000194, 0.1499999999999999944, 0.2000000000000000389, 0.2500000000000000000, 0.2999999999999999889, 0.3499999999999999223, 0.4000000000000000777 ),
 .UNSPECIFIED. ) 
 CURVE ( )  GEOMETRIC_REPRESENTATION_ITEM ( )  RATIONAL_B_SPLINE_CURVE ( ( 1.000000000000000000, 0.9876883405951377704, 1.000000000000000000, 0.9876883405951377704, 1.000000000000000000, 0.9876883405951377704, 1.000000000000000000, 0.9876883405951377704, 1.000000000000000000, 0.9876883405951377704, 1.000000000000000000, 0.9876883405951377704, 1.000000000000000000, 0.9876883405951377704, 1.000000000000000000, 0.9876883405951377704, 1.000000000000000000 ) ) 
 REPRESENTATION_ITEM ( '' )  );
#11027=ORIENTED_EDGE ( 'NONE', *, *, #10679, .F. ) ;
#11030=LINE ( 'NONE', #9535, #880 ) ;
#11036=CARTESIAN_POINT ( 'NONE',  ( 3.270778111535314281, -3.632567103900546712, -12.84374999795161543 ) ) ;
#11054=CARTESIAN_POINT ( 'NONE',  ( -4.936344801571327601, -2.849999999999954792, -11.00000000000000711 ) ) ;
#11082=CARTESIAN_POINT ( 'NONE',  ( -2.993098736590125853E-16, 4.888101187500000222, -11.46874999795161543 ) ) ;
#11087=CIRCLE ( 'NONE', #17487, 4.200000000000001954 ) ;
#11095=CARTESIAN_POINT ( 'NONE',  ( 4.080749450109621534, -4.080749450109678378, -8.500000000000007105 ) ) ;
#11101=CARTESIAN_POINT ( 'NONE',  ( 5.668774803599156975, -0.5958122406256377568, -13.00000000000000533 ) ) ;
#11131=CARTESIAN_POINT ( 'NONE',  ( 1.493657965219485462, -5.574407415329169169, -14.81249999590322375 ) ) ;
#11134=CARTESIAN_POINT ( 'NONE',  ( -4.780397808154247308, 1.280903732194486722, -14.34374999795161365 ) ) ;
#11137=CARTESIAN_POINT ( 'NONE',  ( 1.988169868018562880, -4.465502636338038123, -13.46874999795161543 ) ) ;
#11144=( BOUNDED_SURFACE ( )  B_SPLINE_SURFACE ( 1, 2, ( 
 ( #9820, #16115, #13200, #19007, #11406, #1093, #11598, #10106, #16208, #2482, #19390, #2577, #16299, #11314, #2391, #19099, #10203 ),
 ( #15912, #7168, #8595, #14412, #13291, #8505, #2193, #3797, #6073, #10694, #19486, #1487, #12189, #15299, #2981, #9095, #7472 ) ),
 .UNSPECIFIED., .F., .F., .F. ) 
 B_SPLINE_SURFACE_WITH_KNOTS ( ( 2, 2 ),
 ( 3, 2, 2, 2, 2, 2, 2, 2, 3 ),
 ( 0.000000000000000000, 1.000000000000000000 ),
 ( 0.000000000000000000, 0.05000000000000000278, 0.1000000000000000056, 0.1499999999999999944, 0.2000000000000000111, 0.2500000000000000000, 0.2999999999999999889, 0.3499999999999999778, 0.4000000000000000222 ),
 .UNSPECIFIED. ) 
 GEOMETRIC_REPRESENTATION_ITEM ( )  RATIONAL_B_SPLINE_SURFACE ( (
 ( 1.000000000000000000, 0.9876883405951377704, 1.000000000000000000, 0.9876883405951377704, 1.000000000000000000, 0.9876883405951377704, 1.000000000000000000, 0.9876883405951377704, 1.000000000000000000, 0.9876883405951377704, 1.000000000000000000, 0.9876883405951377704, 1.000000000000000000, 0.9876883405951377704, 1.000000000000000000, 0.9876883405951377704, 1.000000000000000000),
 ( 1.000000000000000000, 0.9876883405951377704, 1.000000000000000000, 0.9876883405951377704, 1.000000000000000000, 0.9876883405951377704, 1.000000000000000000, 0.9876883405951377704, 1.000000000000000000, 0.9876883405951377704, 1.000000000000000000, 0.9876883405951377704, 1.000000000000000000, 0.9876883405951377704, 1.000000000000000000, 0.9876883405951377704, 1.000000000000000000) ) ) 
 REPRESENTATION_ITEM ( '' )  SURFACE ( )  );
#11180=CARTESIAN_POINT ( 'NONE',  ( -3.814044456245444081, 4.235925505221192822, -12.00000000000000533 ) ) ;
#11181=MECHANICAL_DESIGN_GEOMETRIC_PRESENTATION_REPRESENTATION('',(#12465),#15665);
#11183=CARTESIAN_POINT ( 'NONE',  ( -5.142044285764750811, 2.620002426024544029, -7.500000000000005329 ) ) ;
#11186=CARTESIAN_POINT ( 'NONE',  ( 2.850000000000024070, 4.936344801571289409, -6.000000000000005329 ) ) ;
#11195=CARTESIAN_POINT ( 'NONE',  ( -3.954556930911881096, -2.873153789725797935, -14.46874999795161720 ) ) ;
#11198=CARTESIAN_POINT ( 'NONE',  ( -1.185096637661215535, 5.575441324182696334, -8.312499995903225525 ) ) ;
#11214=ORIENTED_EDGE ( 'NONE', *, *, #6593, .T. ) ;
#11221=CARTESIAN_POINT ( 'NONE',  ( -3.814044456245444081, 4.235925505221192822, -13.31249999590322730 ) ) ;
#11225=CARTESIAN_POINT ( 'NONE',  ( 5.700000000000001954, 0.000000000000000000, 0.000000000000000000 ) ) ;
#11242=CARTESIAN_POINT ( 'NONE',  ( 2.444050593749960587, -4.233219804643904460, -6.468749997951615427 ) ) ;
#11269=CARTESIAN_POINT ( 'NONE',  ( -1.493657965219562511, -5.574407415329147852, -8.500000000000005329 ) ) ;
#11274=ORIENTED_EDGE ( 'NONE', *, *, #7324, .F. ) ;
#11278=VERTEX_POINT ( 'NONE', #8085 ) ;
#11301=DIRECTION ( 'NONE',  ( -0.000000000000000000, -0.000000000000000000, 1.000000000000000000 ) ) ;
#11305=LINE ( 'NONE', #17405, #9866 ) ;
#11314=CARTESIAN_POINT ( 'NONE',  ( 2.620002426024544029, 5.142044285764750811, -13.81249999590322552 ) ) ;
#11320=CARTESIAN_POINT ( 'NONE',  ( -4.200000000000000178, 5.143516556418885886E-16, -28.99999999999999645 ) ) ;
#11328=AXIS2_PLACEMENT_3D ( 'NONE', #12560, #7745, #17353 ) ;
#11340=CARTESIAN_POINT ( 'NONE',  ( 2.695436003842704764, -4.150607464521812062, -13.34374999795161365 ) ) ;
#11354=CARTESIAN_POINT ( 'NONE',  ( 5.142044285764733935, -2.620002426024580000, -7.500000000000005329 ) ) ;
#11369=CARTESIAN_POINT ( 'NONE',  ( -1.988169868018530906, 4.465502636338051445, -13.84374999795161543 ) ) ;
#11395=CARTESIAN_POINT ( 'NONE',  ( -0.7741991708319226895, -4.888101187499994893, -11.96874999795161365 ) ) ;
#11406=CARTESIAN_POINT ( 'NONE',  ( -4.611396867937201272, 3.350375938067097437, -9.312499995903225525 ) ) ;
#11408=ORIENTED_EDGE ( 'NONE', *, *, #16681, .F. ) ;
#11421=VECTOR ( 'NONE', #13978, 1000.000000000000000 ) ;
#11426=ORIENTED_EDGE ( 'NONE', *, *, #7008, .T. ) ;
#11431=ADVANCED_FACE ( 'NONE', ( #980 ), #17887, .F. ) ;
#11437=CARTESIAN_POINT ( 'NONE',  ( 1.773574444220693103, -4.620319390059841602, -7.343749997951615427 ) ) ;
#11445=CARTESIAN_POINT ( 'NONE',  ( 4.888101187499994893, -0.7741991708319229115, -7.343749997951615427 ) ) ;
#11448=CARTESIAN_POINT ( 'NONE',  ( 3.350375938067065462, -4.611396867937225252, -9.000000000000005329 ) ) ;
#11461=CARTESIAN_POINT ( 'NONE',  ( -5.700000000000001066, 0.000000000000000000, -6.000000000000005329 ) ) ;
#11471=ORIENTED_EDGE ( 'NONE', *, *, #12016, .F. ) ;
#11472=CARTESIAN_POINT ( 'NONE',  ( -4.781284448697179279, 1.016293382781477961, -10.84374999795161543 ) ) ;
#11477=CARTESIAN_POINT ( 'NONE',  ( -1.988169868018530906, 4.465502636338051445, -13.46874999795161543 ) ) ;
#11485=EDGE_CURVE ( 'NONE', #11735, #17426, #4576, .T. ) ;
#11502=CARTESIAN_POINT ( 'NONE',  ( 1.773574444220693103, -4.620319390059842490, -7.343749997951615427 ) ) ;
#11536=CARTESIAN_POINT ( 'NONE',  ( -1.510506337161893642, -4.648860486681943627, -12.84374999795161543 ) ) ;
#11539=CARTESIAN_POINT ( 'NONE',  ( -3.499494075959840078, -3.499494075959792116, -13.96874999795161365 ) ) ;
#11549=( BOUNDED_CURVE ( )  B_SPLINE_CURVE ( 2, ( #16908, #1888, #18789, #4892, #7788, #3392, #1696, #12795, #7880 ),
 .UNSPECIFIED., .F., .F. ) 
 B_SPLINE_CURVE_WITH_KNOTS ( ( 3, 2, 2, 2, 3 ),
 ( 0.000000000000000000, 0.05000000000000000278, 0.1000000000000000056, 0.1499999999999999944, 0.1666819079834106210 ),
 .UNSPECIFIED. ) 
 CURVE ( )  GEOMETRIC_REPRESENTATION_ITEM ( )  RATIONAL_B_SPLINE_CURVE ( ( 1.000000000000000000, 0.9876883405951377704, 1.000000000000000000, 0.9876883405951377704, 1.000000000000000000, 0.9876883405951377704, 1.000000000000000000, 0.9958923606136999007, 0.9945256517182514688 ) ) 
 REPRESENTATION_ITEM ( '' )  );
#11557=CARTESIAN_POINT ( 'NONE',  ( -5.294050593750000644, 0.000000000000000000, -6.234374998975811266 ) ) ;
#11565=CARTESIAN_POINT ( 'NONE',  ( -2.695436003842674566, 4.150607464521828938, -12.96874999795161543 ) ) ;
#11566=CARTESIAN_POINT ( 'NONE',  ( -1.773574444220725077, 4.620319390059829168, -6.968749997951614539 ) ) ;
#11570=CARTESIAN_POINT ( 'NONE',  ( -3.270778111535288080, 3.632567103900569361, -12.46874999795161543 ) ) ;
#11596=CARTESIAN_POINT ( 'NONE',  ( 5.575441324182689229, -1.185096637661254171, -11.31249999590322375 ) ) ;
#11598=CARTESIAN_POINT ( 'NONE',  ( -3.350375938067097437, 4.611396867937201272, -10.31249999590322552 ) ) ;
#11622=CARTESIAN_POINT ( 'NONE',  ( -0.5109457054261112852, 4.861323657744413218, -14.84374999795161543 ) ) ;
#11635=CARTESIAN_POINT ( 'NONE',  ( 2.873153789725797491, -3.954556930911881985, -9.468749997951615427 ) ) ;
#11649=EDGE_CURVE ( 'NONE', #19556, #19358, #11087, .T. ) ;
#11660=( BOUNDED_CURVE ( )  B_SPLINE_CURVE ( 2, ( #17175, #3464, #3260, #12771, #6441, #11269, #571, #6643, #7856, #12577, #9574, #1959, #5150, #10972, #17076 ),
 .UNSPECIFIED., .F., .F. ) 
 B_SPLINE_CURVE_WITH_KNOTS ( ( 3, 2, 2, 2, 2, 2, 2, 3 ),
 ( 0.000000000000000000, 0.05000000000000000278, 0.1000000000000000056, 0.1499999999999999944, 0.2000000000000000111, 0.2500000000000000000, 0.2999999999999999889, 0.3333180920165860761 ),
 .UNSPECIFIED. ) 
 CURVE ( )  GEOMETRIC_REPRESENTATION_ITEM ( )  RATIONAL_B_SPLINE_CURVE ( ( 1.000000000000000000, 0.9876883405951377704, 1.000000000000000000, 0.9876883405951377704, 1.000000000000000000, 0.9876883405951377704, 1.000000000000000000, 0.9876883405951377704, 1.000000000000000000, 0.9876883405951377704, 1.000000000000000000, 0.9876883405951377704, 1.000000000000000000, 0.9917959799814386468, 0.9945256517182510247 ) ) 
 REPRESENTATION_ITEM ( '' )  );
#11661=CARTESIAN_POINT ( 'NONE',  ( -4.861323657744413218, -0.5109457054261099529, -9.468749997951615427 ) ) ;
#11674=CARTESIAN_POINT ( 'NONE',  ( 0.5958122406255995651, -5.668774803599162304, -15.31249999590322552 ) ) ;
#11686=ORIENTED_EDGE ( 'NONE', *, *, #1103, .F. ) ;
#11693=CARTESIAN_POINT ( 'NONE',  ( 2.695436003842704764, -4.150607464521811174, -12.96874999795161543 ) ) ;
#11694=CARTESIAN_POINT ( 'NONE',  ( -4.942249507334558700, -0.2590123213420630899, -13.34374999795161365 ) ) ;
#11698=ORIENTED_EDGE ( 'NONE', *, *, #14856, .T. ) ;
#11711=B_SPLINE_CURVE_WITH_KNOTS ( 'NONE', 1,
 ( #5563, #11674 ),
 .UNSPECIFIED., .F., .F.,
 ( 2, 2 ),
 ( 0.000000000000000000, 1.000000000000000000 ),
 .UNSPECIFIED. ) ;
#11719=CARTESIAN_POINT ( 'NONE',  ( -3.954556930911881096, -2.873153789725797935, -14.46874999795161720 ) ) ;
#11720=CARTESIAN_POINT ( 'NONE',  ( -4.080749450109650844, 4.080749450109650844, -8.500000000000005329 ) ) ;
#11722=CARTESIAN_POINT ( 'NONE',  ( 1.773574444220693103, -4.620319390059841602, -6.968749997951614539 ) ) ;
#11730=CARTESIAN_POINT ( 'NONE',  ( -2.873153789725852558, -3.954556930911842016, -13.84374999795161543 ) ) ;
#11732=CARTESIAN_POINT ( 'NONE',  ( -2.444050593749990341, 4.233219804643887585, -6.843749997951615427 ) ) ;
#11735=VERTEX_POINT ( 'NONE', #17180 ) ;
#11762=CARTESIAN_POINT ( 'NONE',  ( 2.647025296874957689, -4.584782303107616031, -6.234374998975811266 ) ) ;
#11771=CARTESIAN_POINT ( 'NONE',  ( 5.387740456496233676, 2.068159791354183596, -11.50000000000000355 ) ) ;
#11791=B_SPLINE_CURVE_WITH_KNOTS ( 'NONE', 1,
 ( #16322, #12015 ),
 .UNSPECIFIED., .F., .F.,
 ( 2, 2 ),
 ( 0.000000000000000000, 1.000000000000000000 ),
 .UNSPECIFIED. ) ;
#11809=CARTESIAN_POINT ( 'NONE',  ( 4.861323657744411442, 0.5109457054261445919, -9.843749997951615427 ) ) ;
#11820=CARTESIAN_POINT ( 'NONE',  ( -3.846120219227966430, -3.114526743279228072, -11.34374999795161543 ) ) ;
#11826=CARTESIAN_POINT ( 'NONE',  ( -4.611396867937224364, -3.350375938067065906, -15.31249999590322552 ) ) ;
#11839=DIRECTION ( 'NONE',  ( -0.000000000000000000, -0.000000000000000000, 1.000000000000000000 ) ) ;
#11849=ADVANCED_FACE ( 'NONE', ( #19731 ), #15342, .F. ) ;
#11859=CARTESIAN_POINT ( 'NONE',  ( -1.988169868018624609, -4.465502636338009701, -9.468749997951615427 ) ) ;
#11868=CARTESIAN_POINT ( 'NONE',  ( 3.814044456245502701, 4.235925505221138643, -10.00000000000000533 ) ) ;
#11919=EDGE_CURVE ( 'NONE', #6321, #1899, #5662, .T. ) ;
#11924=VECTOR ( 'NONE', #18060, 1000.000000000000000 ) ;
#11929=CARTESIAN_POINT ( 'NONE',  ( -2.444050593749990341, 4.233219804643887585, -6.468749997951615427 ) ) ;
#11938=( NAMED_UNIT ( * ) SI_UNIT ( $, .STERADIAN. ) SOLID_ANGLE_UNIT ( ) );
#11941=CARTESIAN_POINT ( 'NONE',  ( 3.954556930911842016, -2.873153789725853002, -8.468749997951615427 ) ) ;
#11962=CARTESIAN_POINT ( 'NONE',  ( -4.780397808154247308, 1.280903732194486722, -13.96874999795161365 ) ) ;
#11963=CARTESIAN_POINT ( 'NONE',  ( 2.068159791354145849, -5.387740456496247887, -7.812499995903224637 ) ) ;
#11972=DIRECTION ( 'NONE',  ( 0.9135454576425977580, -0.4067366430758074247, 0.000000000000000000 ) ) ;
#11992=DIRECTION ( 'NONE',  ( -0.000000000000000000, -0.000000000000000000, 1.000000000000000000 ) ) ;
#12013=DIRECTION ( 'NONE',  ( -0.000000000000000000, -0.000000000000000000, 1.000000000000000000 ) ) ;
#12015=CARTESIAN_POINT ( 'NONE',  ( 4.611396867937200383, 3.350375938067097881, -15.31249999590322552 ) ) ;
#12016=EDGE_CURVE ( 'NONE', #1514, #12259, #6796, .T. ) ;
#12019=EDGE_CURVE ( 'NONE', #2597, #1514, #11030, .T. ) ;
#12022=CARTESIAN_POINT ( 'NONE',  ( 4.781284448697195266, 1.016293382781411792, -12.84374999795161543 ) ) ;
#12027=VERTEX_POINT ( 'NONE', #18530 ) ;
#12029=CARTESIAN_POINT ( 'NONE',  ( 2.873153789725825025, 3.954556930911862000, -13.46874999795161543 ) ) ;
#12030=CARTESIAN_POINT ( 'NONE',  ( 4.888101187500000222, -3.413342815706642518E-14, -6.843749997951615427 ) ) ;
#12033=CARTESIAN_POINT ( 'NONE',  ( 2.695436003842732298, 4.150607464521791634, -10.34374999795161543 ) ) ;
#12072=CARTESIAN_POINT ( 'NONE',  ( 1.493657965219523875, 5.574407415329156734, -9.812499995903223748 ) ) ;
#12100=CARTESIAN_POINT ( 'NONE',  ( -1.280903732194386802, 4.780397808154273065, -13.96874999795161365 ) ) ;
#12109=CYLINDRICAL_SURFACE ( 'NONE', #859, 5.700000000000001954 ) ;
#12123=CARTESIAN_POINT ( 'NONE',  ( -4.465502636338010589, 1.988169868018623720, -14.46874999795161720 ) ) ;
#12128=CARTESIAN_POINT ( 'NONE',  ( -1.510506337161861667, 4.648860486681953397, -10.84374999795161543 ) ) ;
#12130=EDGE_CURVE ( 'NONE', #13685, #8919, #15931, .T. ) ;
#12133=FACE_OUTER_BOUND ( 'NONE', #17240, .T. ) ;
#12142=SURFACE_STYLE_USAGE ( .BOTH. , #4336 ) ;
#12166=ORIENTED_EDGE ( 'NONE', *, *, #2684, .F. ) ;
#12174=CARTESIAN_POINT ( 'NONE',  ( 0.5109457054261454800, -4.861323657744410554, -14.46874999795161720 ) ) ;
#12180=CARTESIAN_POINT ( 'NONE',  ( 9.000000000000001776, 0.000000000000000000, 0.000000000000000000 ) ) ;
#12189=CARTESIAN_POINT ( 'NONE',  ( 1.510506337161861223, 4.648860486681953397, -12.84374999795161543 ) ) ;
#12195=CYLINDRICAL_SURFACE ( 'NONE', #18738, 9.000000000000001776 ) ;
#12198=CARTESIAN_POINT ( 'NONE',  ( -5.574407415329146964, 1.493657965219562067, -14.81249999590322375 ) ) ;
#12207=CARTESIAN_POINT ( 'NONE',  ( 0.5109457054261454800, -4.861323657744410554, -14.84374999795161543 ) ) ;
#12219=CARTESIAN_POINT ( 'NONE',  ( 3.846120219227944670, 3.114526743279256049, -11.34374999795161543 ) ) ;
#12236=EDGE_CURVE ( 'NONE', #12259, #6178, #10324, .T. ) ;
#12254=DIRECTION ( 'NONE',  ( -0.8660254037844363761, 0.5000000000000039968, 0.000000000000000000 ) ) ;
#12258=CARTESIAN_POINT ( 'NONE',  ( 4.620319390059819398, -1.773574444220757274, -10.96874999795161720 ) ) ;
#12259=VERTEX_POINT ( 'NONE', #19611 ) ;
#12260=CARTESIAN_POINT ( 'NONE',  ( -1.773574444220725077, 4.620319390059829168, -6.968749997951614539 ) ) ;
#12268=CARTESIAN_POINT ( 'NONE',  ( -2.444050593749990785, 4.233219804643887585, -6.843749997951615427 ) ) ;
#12280=CARTESIAN_POINT ( 'NONE',  ( 0.9027913098498173694, -5.700000000000006395, -11.81249999590322552 ) ) ;
#12295=CARTESIAN_POINT ( 'NONE',  ( -0.9027913098498572264, 5.699999999999999289, -10.50000000000000711 ) ) ;
#12306=EDGE_LOOP ( 'NONE', ( #19730, #13542, #6561, #1633 ) ) ;
#12315=( BOUNDED_SURFACE ( )  B_SPLINE_SURFACE ( 1, 2, ( 
 ( #14464, #12962, #12860, #18956, #19055, #5247, #5344, #17560, #3847, #8741, #14659, #7123, #8941, #19531, #5826, #1235, #8844 ),
 ( #3947, #13338, #19244, #13539, #11941, #13253, #4339, #14943, #7315, #17656, #14751, #8644, #5630, #18052, #947, #19641, #1144 ) ),
 .UNSPECIFIED., .F., .F., .F. ) 
 B_SPLINE_SURFACE_WITH_KNOTS ( ( 2, 2 ),
 ( 3, 2, 2, 2, 2, 2, 2, 2, 3 ),
 ( 0.000000000000000000, 1.000000000000000000 ),
 ( 0.000000000000000000, 0.05000000000000000278, 0.1000000000000000056, 0.1499999999999999944, 0.2000000000000000111, 0.2500000000000000000, 0.2999999999999999889, 0.3499999999999999778, 0.4000000000000000222 ),
 .UNSPECIFIED. ) 
 GEOMETRIC_REPRESENTATION_ITEM ( )  RATIONAL_B_SPLINE_SURFACE ( (
 ( 1.000000000000000000, 0.9876883405951377704, 1.000000000000000000, 0.9876883405951377704, 1.000000000000000000, 0.9876883405951377704, 1.000000000000000000, 0.9876883405951377704, 1.000000000000000000, 0.9876883405951377704, 1.000000000000000000, 0.9876883405951377704, 1.000000000000000000, 0.9876883405951377704, 1.000000000000000000, 0.9876883405951377704, 1.000000000000000000),
 ( 1.000000000000000000, 0.9876883405951377704, 1.000000000000000000, 0.9876883405951377704, 1.000000000000000000, 0.9876883405951377704, 1.000000000000000000, 0.9876883405951377704, 1.000000000000000000, 0.9876883405951377704, 1.000000000000000000, 0.9876883405951377704, 1.000000000000000000, 0.9876883405951377704, 1.000000000000000000, 0.9876883405951377704, 1.000000000000000000) ) ) 
 REPRESENTATION_ITEM ( '' )  SURFACE ( )  );
#12320=ORIENTED_EDGE ( 'NONE', *, *, #12772, .T. ) ;
#12330=DIRECTION ( 'NONE',  ( 0.4330127018922180770, -0.7500000000000021094, 0.4999999999999979461 ) ) ;
#12331=CARTESIAN_POINT ( 'NONE',  ( 4.888101187499994893, -0.7741991708319229115, -7.343749997951615427 ) ) ;
#12339=DIRECTION ( 'NONE',  ( 1.000000000000000000, 0.000000000000000000, 0.000000000000000000 ) ) ;
#12353=DIRECTION ( 'NONE',  ( -0.5000000000000039968, -0.8660254037844363761, 0.000000000000000000 ) ) ;
#12354=CARTESIAN_POINT ( 'NONE',  ( -0.5958122406255600412, 5.668774803599166745, 0.000000000000000000 ) ) ;
#12359=ADVANCED_FACE ( 'NONE', ( #18798, #6188 ), #14200, .F. ) ;
#12366=ORIENTED_EDGE ( 'NONE', *, *, #9471, .T. ) ;
#12370=CARTESIAN_POINT ( 'NONE',  ( -0.3020334839682480288, 5.763142191869157216, -8.812499995903225525 ) ) ;
#12380=EDGE_CURVE ( 'NONE', #2597, #12952, #5519, .T. ) ;
#12384=CARTESIAN_POINT ( 'NONE',  ( 5.700000000000001066, -4.360680574150373717E-16, -12.66727757604273386 ) ) ;
#12388=CARTESIAN_POINT ( 'NONE',  ( -5.763142191869158992, -0.3020334839682081163, -13.81249999590322552 ) ) ;
#12410=LINE ( 'NONE', #9605, #8322 ) ;
#12414=CARTESIAN_POINT ( 'NONE',  ( 5.575441324182689229, -1.185096637661254171, -10.00000000000000533 ) ) ;
#12421=CARTESIAN_POINT ( 'NONE',  ( 0.000000000000000000, 0.000000000000000000, 0.000000000000000000 ) ) ;
#12428=DIRECTION ( 'NONE',  ( 0.000000000000000000, 0.000000000000000000, 1.000000000000000000 ) ) ;
#12431=LINE ( 'NONE', #529, #3522 ) ;
#12434=CARTESIAN_POINT ( 'NONE',  ( 5.575441324182689229, -1.185096637661254171, -11.31249999590322375 ) ) ;
#12435=ORIENTED_EDGE ( 'NONE', *, *, #15249, .F. ) ;
#12437=CARTESIAN_POINT ( 'NONE',  ( -0.5109457054262123155, -4.861323657744403448, -8.843749997951615427 ) ) ;
#12438=CARTESIAN_POINT ( 'NONE',  ( -3.631840208645857437, -4.484949146646330931, -6.500000000000005329 ) ) ;
#12453=ORIENTED_EDGE ( 'NONE', *, *, #13163, .F. ) ;
#12463=CARTESIAN_POINT ( 'NONE',  ( 4.861323657744407001, -0.5109457054261775655, -13.84374999795161543 ) ) ;
#12465=STYLED_ITEM ( 'NONE', ( #15346 ), #16364 ) ;
#12471=DIRECTION ( 'NONE',  ( 0.000000000000000000, -0.000000000000000000, -1.000000000000000000 ) ) ;
#12481=CARTESIAN_POINT ( 'NONE',  ( 2.849999999999954348, -4.936344801571327601, -7.312499995903225525 ) ) ;
#12487=CARTESIAN_POINT ( 'NONE',  ( 4.611396867937200383, 3.350375938067097881, -14.00000000000000533 ) ) ;
#12505=CARTESIAN_POINT ( 'NONE',  ( 5.574407415329157622, -1.493657965219523209, -13.50000000000000533 ) ) ;
#12507=CARTESIAN_POINT ( 'NONE',  ( -2.444050593750049849, -4.233219804643852946, -6.656249997951614539 ) ) ;
#12516=CARTESIAN_POINT ( 'NONE',  ( -1.510506337161861667, 4.648860486681953397, -10.84374999795161543 ) ) ;
#12524=VECTOR ( 'NONE', #7698, 1000.000000000000000 ) ;
#12529=CARTESIAN_POINT ( 'NONE',  ( 0.7741991708318884946, 4.888101187500000222, -11.96874999795161365 ) ) ;
#12531=DIRECTION ( 'NONE',  ( -0.000000000000000000, -0.000000000000000000, 1.000000000000000000 ) ) ;
#12534=DIRECTION ( 'NONE',  ( -0.000000000000000000, -0.000000000000000000, 1.000000000000000000 ) ) ;
#12549=( BOUNDED_SURFACE ( )  B_SPLINE_SURFACE ( 1, 2, ( 
 ( #7437, #17866, #19661, #7232, #13357, #7332, #11859, #13452, #17970, #4260, #5846, #10372, #19553, #16470, #14964, #11962, #18068 ),
 ( #4359, #10468, #2848, #10959, #4849, #3450, #10858, #1942, #17064, #5046, #11054, #1653, #12564, #1554, #17160, #18750, #6143 ) ),
 .UNSPECIFIED., .F., .F., .F. ) 
 B_SPLINE_SURFACE_WITH_KNOTS ( ( 2, 2 ),
 ( 3, 2, 2, 2, 2, 2, 2, 2, 3 ),
 ( 0.000000000000000000, 1.000000000000000000 ),
 ( 0.000000000000000000, 0.05000000000000000278, 0.1000000000000000056, 0.1499999999999999944, 0.2000000000000000111, 0.2500000000000000000, 0.2999999999999999889, 0.3499999999999999778, 0.4000000000000000222 ),
 .UNSPECIFIED. ) 
 GEOMETRIC_REPRESENTATION_ITEM ( )  RATIONAL_B_SPLINE_SURFACE ( (
 ( 1.000000000000000000, 0.9876883405951377704, 1.000000000000000000, 0.9876883405951377704, 1.000000000000000000, 0.9876883405951377704, 1.000000000000000000, 0.9876883405951377704, 1.000000000000000000, 0.9876883405951377704, 1.000000000000000000, 0.9876883405951377704, 1.000000000000000000, 0.9876883405951377704, 1.000000000000000000, 0.9876883405951377704, 1.000000000000000000),
 ( 1.000000000000000000, 0.9876883405951377704, 1.000000000000000000, 0.9876883405951377704, 1.000000000000000000, 0.9876883405951377704, 1.000000000000000000, 0.9876883405951377704, 1.000000000000000000, 0.9876883405951377704, 1.000000000000000000, 0.9876883405951377704, 1.000000000000000000, 0.9876883405951377704, 1.000000000000000000, 0.9876883405951377704, 1.000000000000000000) ) ) 
 REPRESENTATION_ITEM ( '' )  SURFACE ( )  );
#12560=CARTESIAN_POINT ( 'NONE',  ( 0.000000000000000000, 0.000000000000000000, 0.000000000000000000 ) ) ;
#12564=CARTESIAN_POINT ( 'NONE',  ( -5.575441324182703440, -1.185096637661177343, -12.00000000000000533 ) ) ;
#12577=CARTESIAN_POINT ( 'NONE',  ( -4.484949146646406426, -3.631840208645763735, -10.50000000000000533 ) ) ;
#12588=CARTESIAN_POINT ( 'NONE',  ( 2.620002426024544029, 5.142044285764750811, -12.50000000000000533 ) ) ;
#12598=EDGE_CURVE ( 'NONE', #736, #9247, #11305, .T. ) ;
#12603=CARTESIAN_POINT ( 'NONE',  ( 2.873153789725797491, -3.954556930911881985, -9.468749997951615427 ) ) ;
#12639=AXIS2_PLACEMENT_3D ( 'NONE', #14500, #12989, #19082 ) ;
#12640=CARTESIAN_POINT ( 'NONE',  ( 3.846120219227923798, -3.114526743279282250, -11.96874999795161365 ) ) ;
#12647=CARTESIAN_POINT ( 'NONE',  ( -3.954556930911881096, -2.873153789725797935, -14.46874999795161720 ) ) ;
#12665=CARTESIAN_POINT ( 'NONE',  ( 0.000000000000000000, 0.000000000000000000, -18.00000000000000355 ) ) ;
#12668=( BOUNDED_CURVE ( )  B_SPLINE_CURVE ( 2, ( #11242, #14246, #6718, #9551, #3635, #4838, #14143, #15847, #5233, #3343, #17346, #5128, #15749, #9758, #18842, #8338, #6618 ),
 .UNSPECIFIED., .F., .F. ) 
 B_SPLINE_CURVE_WITH_KNOTS ( ( 3, 2, 2, 2, 2, 2, 2, 2, 3 ),
 ( 0.000000000000000000, 0.05000000000000000971, 0.1000000000000000194, 0.1499999999999999944, 0.2000000000000000389, 0.2500000000000000000, 0.2999999999999999889, 0.3499999999999999223, 0.4000000000000000777 ),
 .UNSPECIFIED. ) 
 CURVE ( )  GEOMETRIC_REPRESENTATION_ITEM ( )  RATIONAL_B_SPLINE_CURVE ( ( 1.000000000000000000, 0.9876883405951377704, 1.000000000000000000, 0.9876883405951377704, 1.000000000000000000, 0.9876883405951377704, 1.000000000000000000, 0.9876883405951377704, 1.000000000000000000, 0.9876883405951377704, 1.000000000000000000, 0.9876883405951377704, 1.000000000000000000, 0.9876883405951377704, 1.000000000000000000, 0.9876883405951377704, 1.000000000000000000 ) ) 
 REPRESENTATION_ITEM ( '' )  );
#12683=CARTESIAN_POINT ( 'NONE',  ( -4.233219804643852946, 2.444050593750049405, -11.46874999795161543 ) ) ;
#12685=CARTESIAN_POINT ( 'NONE',  ( -3.632567103900569361, -3.270778111535287191, -7.843749997951614539 ) ) ;
#12716=CARTESIAN_POINT ( 'NONE',  ( -5.207209108562804722, 2.318398865532109276, -14.00000000000000533 ) ) ;
#12721=CARTESIAN_POINT ( 'NONE',  ( 2.444050593749960587, -4.233219804643904460, -6.656249997951614539 ) ) ;
#12771=CARTESIAN_POINT ( 'NONE',  ( 0.3020334839682081163, -5.763142191869158992, -7.500000000000005329 ) ) ;
#12772=EDGE_CURVE ( 'NONE', #12027, #5242, #2672, .T. ) ;
#12781=CARTESIAN_POINT ( 'NONE',  ( -4.942249507334553371, 0.2590123213421660631, -9.968749997951617203 ) ) ;
#12795=CARTESIAN_POINT ( 'NONE',  ( -5.700000000000001066, -0.2987243419133009947, -10.47794484381773650 ) ) ;
#12797=CARTESIAN_POINT ( 'NONE',  ( 4.409619785863891472, -2.246813503491864150, -7.968749997951616315 ) ) ;
#12811=ORIENTED_EDGE ( 'NONE', *, *, #51, .T. ) ;
#12818=DIRECTION ( 'NONE',  ( 0.000000000000000000, 0.000000000000000000, 1.000000000000000000 ) ) ;
#12826=ORIENTED_EDGE ( 'NONE', *, *, #8714, .F. ) ;
#12833=CARTESIAN_POINT ( 'NONE',  ( 4.465502636338039011, 1.988169868018562436, -8.843749997951615427 ) ) ;
#12845=VERTEX_POINT ( 'NONE', #12481 ) ;
#12853=VERTEX_POINT ( 'NONE', #4874 ) ;
#12859=ORIENTED_EDGE ( 'NONE', *, *, #4890, .T. ) ;
#12860=CARTESIAN_POINT ( 'NONE',  ( 4.648860486681943627, -1.510506337161893864, -7.843749997951614539 ) ) ;
#12863=CARTESIAN_POINT ( 'NONE',  ( -4.465502636338051445, -1.988169868018530462, -8.843749997951615427 ) ) ;
#12880=CARTESIAN_POINT ( 'NONE',  ( -0.5958122406255597081, 5.668774803599165857, -14.00000000000000533 ) ) ;
#12895=CARTESIAN_POINT ( 'NONE',  ( 3.954556930911842016, -2.873153789725853002, -8.468749997951615427 ) ) ;
#12915=CARTESIAN_POINT ( 'NONE',  ( 9.000000000000001776, 0.000000000000000000, -22.00000000000000000 ) ) ;
#12922=CARTESIAN_POINT ( 'NONE',  ( -3.143139765844555900, 4.840010801796527318, -13.81249999590322730 ) ) ;
#12926=ORIENTED_EDGE ( 'NONE', *, *, #17245, .T. ) ;
#12931=B_SPLINE_CURVE_WITH_KNOTS ( 'NONE', 1,
 ( #5092, #6579 ),
 .UNSPECIFIED., .F., .F.,
 ( 2, 2 ),
 ( 0.000000000000000000, 1.000000000000000000 ),
 .UNSPECIFIED. ) ;
#12936=CARTESIAN_POINT ( 'NONE',  ( -5.142044285764751699, 2.620002426024544029, -7.500000000000005329 ) ) ;
#12950=CARTESIAN_POINT ( 'NONE',  ( -3.383411828340740850E-14, -4.888101187500000222, -11.46874999795161543 ) ) ;
#12952=VERTEX_POINT ( 'NONE', #6755 ) ;
#12954=CIRCLE ( 'NONE', #17103, 9.000000000000001776 ) ;
#12957=DIRECTION ( 'NONE',  ( -0.000000000000000000, -0.000000000000000000, 1.000000000000000000 ) ) ;
#12962=CARTESIAN_POINT ( 'NONE',  ( 4.888101187499994893, -0.7741991708319229115, -7.343749997951615427 ) ) ;
#12965=EDGE_LOOP ( 'NONE', ( #4611, #15808, #10, #347 ) ) ;
#12969=ADVANCED_FACE ( 'NONE', ( #778 ), #8860, .T. ) ;
#12971=CARTESIAN_POINT ( 'NONE',  ( -2.444050593749990785, 4.233219804643887585, -6.843749997951615427 ) ) ;
#12975=CARTESIAN_POINT ( 'NONE',  ( 0.5109457054261784537, 4.861323657744407001, -8.468749997951615427 ) ) ;
#12976=VERTEX_POINT ( 'NONE', #2366 ) ;
#12979=VECTOR ( 'NONE', #13629, 1000.000000000000000 ) ;
#12989=DIRECTION ( 'NONE',  ( -0.000000000000000000, -0.000000000000000000, 1.000000000000000000 ) ) ;
#13005=CARTESIAN_POINT ( 'NONE',  ( 4.484949146646356688, -3.631840208645826351, -12.81249999590322552 ) ) ;
#13029=ORIENTED_EDGE ( 'NONE', *, *, #443, .T. ) ;
#13041=CARTESIAN_POINT ( 'NONE',  ( 5.699999596629369059, -0.002144393866035136480, -6.000593838912648081 ) ) ;
#13044=CARTESIAN_POINT ( 'NONE',  ( 4.611396867937178179, -3.350375938067129855, -8.000000000000005329 ) ) ;
#13046=ORIENTED_EDGE ( 'NONE', *, *, #615, .F. ) ;
#13053=DIRECTION ( 'NONE',  ( 1.000000000000000000, 0.000000000000000000, 0.000000000000000000 ) ) ;
#13097=CARTESIAN_POINT ( 'NONE',  ( 4.620319390059819398, -1.773574444220757274, -11.34374999795161543 ) ) ;
#13100=CARTESIAN_POINT ( 'NONE',  ( 1.016293382781377819, -4.781284448697200595, -7.843749997951614539 ) ) ;
#13109=DIRECTION ( 'NONE',  ( -0.000000000000000000, -0.000000000000000000, 1.000000000000000000 ) ) ;
#13110=DIRECTION ( 'NONE',  ( 0.4999999999999978351, -0.8660254037844398178, 0.000000000000000000 ) ) ;
#13111=DIRECTION ( 'NONE',  ( -0.000000000000000000, -0.000000000000000000, 1.000000000000000000 ) ) ;
#13125=EDGE_CURVE ( 'NONE', #7839, #17369, #2851, .T. ) ;
#13128=ORIENTED_EDGE ( 'NONE', *, *, #13911, .F. ) ;
#13134=CARTESIAN_POINT ( 'NONE',  ( 4.888101187500000222, -3.413342815706642518E-14, -6.843749997951615427 ) ) ;
#13138=CARTESIAN_POINT ( 'NONE',  ( -2.647025296875054057, -4.584782303107560963, -6.234374998975811266 ) ) ;
#13145=FACE_OUTER_BOUND ( 'NONE', #9955, .T. ) ;
#13156=FACE_OUTER_BOUND ( 'NONE', #266, .T. ) ;
#13163=EDGE_CURVE ( 'NONE', #19526, #17330, #16671, .T. ) ;
#13167=CARTESIAN_POINT ( 'NONE',  ( -3.270778111535288080, 3.632567103900569361, -12.84374999795161543 ) ) ;
#13169=CARTESIAN_POINT ( 'NONE',  ( 1.988169868018593300, 4.465502636338023912, -9.468749997951615427 ) ) ;
#13186=( BOUNDED_SURFACE ( )  B_SPLINE_SURFACE ( 1, 2, ( 
 ( #11732, #19725, #10241, #10343, #2715, #5713, #15131, #12033, #18042, #7402, #8928, #15032, #4422, #13240, #5812, #6010, #16334 ),
 ( #11929, #2910, #7302, #1322, #4326, #2616, #13327, #4514, #10631, #13628, #1426, #1224, #17834, #19428, #8730, #13527, #10437 ) ),
 .UNSPECIFIED., .F., .F., .F. ) 
 B_SPLINE_SURFACE_WITH_KNOTS ( ( 2, 2 ),
 ( 3, 2, 2, 2, 2, 2, 2, 2, 3 ),
 ( 0.000000000000000000, 1.000000000000000000 ),
 ( 0.000000000000000000, 0.05000000000000000278, 0.1000000000000000056, 0.1499999999999999944, 0.2000000000000000111, 0.2500000000000000000, 0.2999999999999999889, 0.3499999999999999778, 0.4000000000000000222 ),
 .UNSPECIFIED. ) 
 GEOMETRIC_REPRESENTATION_ITEM ( )  RATIONAL_B_SPLINE_SURFACE ( (
 ( 1.000000000000000000, 0.9876883405951377704, 1.000000000000000000, 0.9876883405951377704, 1.000000000000000000, 0.9876883405951377704, 1.000000000000000000, 0.9876883405951377704, 1.000000000000000000, 0.9876883405951377704, 1.000000000000000000, 0.9876883405951377704, 1.000000000000000000, 0.9876883405951377704, 1.000000000000000000, 0.9876883405951377704, 1.000000000000000000),
 ( 1.000000000000000000, 0.9876883405951377704, 1.000000000000000000, 0.9876883405951377704, 1.000000000000000000, 0.9876883405951377704, 1.000000000000000000, 0.9876883405951377704, 1.000000000000000000, 0.9876883405951377704, 1.000000000000000000, 0.9876883405951377704, 1.000000000000000000, 0.9876883405951377704, 1.000000000000000000, 0.9876883405951377704, 1.000000000000000000) ) ) 
 REPRESENTATION_ITEM ( '' )  SURFACE ( )  );
#13200=CARTESIAN_POINT ( 'NONE',  ( -5.421022142882375938, 1.761396867937200517, -8.312499995903225525 ) ) ;
#13210=CYLINDRICAL_SURFACE ( 'NONE', #7678, 5.700000000000001954 ) ;
#13225=CARTESIAN_POINT ( 'NONE',  ( -3.350375938067097437, 4.611396867937201272, -10.31249999590322552 ) ) ;
#13231=CARTESIAN_POINT ( 'NONE',  ( -3.270778111535363131, -3.632567103900500971, -10.84374999795161543 ) ) ;
#13240=CARTESIAN_POINT ( 'NONE',  ( 4.942249507334556924, 0.2590123213420971182, -13.34374999795161365 ) ) ;
#13241=CARTESIAN_POINT ( 'NONE',  ( 2.620002426024508502, -5.142044285764769462, -9.500000000000005329 ) ) ;
#13253=CARTESIAN_POINT ( 'NONE',  ( 3.499494075959791672, -3.499494075959840966, -8.968749997951611874 ) ) ;
#13257=EDGE_LOOP ( 'NONE', ( #2176, #17879, #1914, #15026 ) ) ;
#13265=CARTESIAN_POINT ( 'NONE',  ( -3.846120219227901593, 3.114526743279308896, -11.96874999795161365 ) ) ;
#13267=CARTESIAN_POINT ( 'NONE',  ( -1.185096637661215091, 5.575441324182695446, -7.000000000000005329 ) ) ;
#13291=CARTESIAN_POINT ( 'NONE',  ( -3.954556930911862000, 2.873153789725825469, -8.843749997951615427 ) ) ;
#13293=VERTEX_POINT ( 'NONE', #15166 ) ;
#13304=CARTESIAN_POINT ( 'NONE',  ( 4.465502636338039011, 1.988169868018562436, -8.843749997951615427 ) ) ;
#13305=EDGE_CURVE ( 'NONE', #9061, #12845, #4855, .T. ) ;
#13327=CARTESIAN_POINT ( 'NONE',  ( 1.988169868018593300, 4.465502636338023912, -9.468749997951615427 ) ) ;
#13337=DIRECTION ( 'NONE',  ( 1.000000000000000000, 0.000000000000000000, 0.000000000000000000 ) ) ;
#13338=CARTESIAN_POINT ( 'NONE',  ( 4.888101187499994893, -0.7741991708319229115, -6.968749997951614539 ) ) ;
#13351=CARTESIAN_POINT ( 'NONE',  ( 4.235925505221166176, 3.814044456245473835, -7.000000000000005329 ) ) ;
#13354=ORIENTED_EDGE ( 'NONE', *, *, #17655, .T. ) ;
#13357=CARTESIAN_POINT ( 'NONE',  ( -0.5109457054262123155, -4.861323657744403448, -8.468749997951615427 ) ) ;
#13366=FACE_OUTER_BOUND ( 'NONE', #16312, .T. ) ;
#13389=FACE_OUTER_BOUND ( 'NONE', #9255, .T. ) ;
#13406=ORIENTED_EDGE ( 'NONE', *, *, #9117, .F. ) ;
#13412=CARTESIAN_POINT ( 'NONE',  ( 5.700000000000001066, 0.000000000000000000, -13.97977757194595760 ) ) ;
#13418=CARTESIAN_POINT ( 'NONE',  ( -3.383411828340740850E-14, -4.888101187500000222, -11.84374999795161365 ) ) ;
#13421=CARTESIAN_POINT ( 'NONE',  ( 5.207209108562838473, 2.318398865532038666, -8.000000000000005329 ) ) ;
#13431=VERTEX_POINT ( 'NONE', #11461 ) ;
#13439=AXIS2_PLACEMENT_3D ( 'NONE', #16906, #3580, #9704 ) ;
#13440=FACE_BOUND ( 'NONE', #16169, .T. ) ;
#13446=CARTESIAN_POINT ( 'NONE',  ( 5.575441324182689229, -1.185096637661254171, -10.00000000000000533 ) ) ;
#13449=CARTESIAN_POINT ( 'NONE',  ( 1.280903732194454303, 4.780397808154257078, -8.968749997951613651 ) ) ;
#13452=CARTESIAN_POINT ( 'NONE',  ( -2.695436003842760275, -4.150607464521772094, -9.968749997951617203 ) ) ;
#13454=VECTOR ( 'NONE', #18051, 1000.000000000000000 ) ;
#13474=ADVANCED_FACE ( 'NONE', ( #6932 ), #12315, .T. ) ;
#13487=CARTESIAN_POINT ( 'NONE',  ( -5.574407415329178939, -1.493657965219446382, -9.812499995903223748 ) ) ;
#13491=DIRECTION ( 'NONE',  ( -0.000000000000000000, -0.000000000000000000, 1.000000000000000000 ) ) ;
#13517=CARTESIAN_POINT ( 'NONE',  ( -4.233219804643904460, -2.444050593749961031, -11.84374999795161365 ) ) ;
#13523=CARTESIAN_POINT ( 'NONE',  ( 2.246813503491833508, 4.409619785863906571, -12.96874999795161543 ) ) ;
#13527=CARTESIAN_POINT ( 'NONE',  ( 4.780397808154257078, -1.280903732194453859, -13.96874999795161365 ) ) ;
#13539=CARTESIAN_POINT ( 'NONE',  ( 4.409619785863891472, -2.246813503491864150, -7.968749997951616315 ) ) ;
#13542=ORIENTED_EDGE ( 'NONE', *, *, #631, .T. ) ;
#13546=PLANE ( 'NONE',  #5892 ) ;
#13553=CARTESIAN_POINT ( 'NONE',  ( 2.695436003842704764, -4.150607464521812062, -12.96874999795161543 ) ) ;
#13556=DIRECTION ( 'NONE',  ( -0.000000000000000000, -0.000000000000000000, 1.000000000000000000 ) ) ;
#13560=CARTESIAN_POINT ( 'NONE',  ( 5.763142191869157216, 0.3020334839682475847, -12.50000000000000533 ) ) ;
#13562=ORIENTED_EDGE ( 'NONE', *, *, #3156, .F. ) ;
#13565=CARTESIAN_POINT ( 'NONE',  ( 2.444050593750020095, 4.233219804643871598, -6.656249997951614539 ) ) ;
#13566=CARTESIAN_POINT ( 'NONE',  ( 0.5109457054261780096, 4.861323657744407001, -8.843749997951615427 ) ) ;
#13578=CARTESIAN_POINT ( 'NONE',  ( -3.945386292505473391E-14, -5.700000000000001066, -12.31249999590322552 ) ) ;
#13595=CARTESIAN_POINT ( 'NONE',  ( -3.270778111535288080, 3.632567103900569361, -12.46874999795161543 ) ) ;
#13609=ORIENTED_EDGE ( 'NONE', *, *, #13125, .F. ) ;
#13612=EDGE_CURVE ( 'NONE', #17046, #1899, #9611, .T. ) ;
#13620=CARTESIAN_POINT ( 'NONE',  ( -4.861323657744403448, 0.5109457054262118714, -13.46874999795161543 ) ) ;
#13624=FACE_OUTER_BOUND ( 'NONE', #9181, .T. ) ;
#13628=CARTESIAN_POINT ( 'NONE',  ( 3.846120219227944670, 3.114526743279255161, -10.96874999795161720 ) ) ;
#13629=DIRECTION ( 'NONE',  ( 0.000000000000000000, 0.000000000000000000, 1.000000000000000000 ) ) ;
#13630=CARTESIAN_POINT ( 'NONE',  ( -9.000000000000000000, 1.102182119232617714E-15, -28.99999999999999645 ) ) ;
#13639=DIRECTION ( 'NONE',  ( 1.000000000000000000, 0.000000000000000000, 0.000000000000000000 ) ) ;
#13654=CARTESIAN_POINT ( 'NONE',  ( 2.318398865532038666, -5.207209108562836697, -13.00000000000000533 ) ) ;
#13662=EDGE_CURVE ( 'NONE', #1899, #13431, #19445, .T. ) ;
#13680=ORIENTED_EDGE ( 'NONE', *, *, #14395, .F. ) ;
#13685=VERTEX_POINT ( 'NONE', #7994 ) ;
#13698=CARTESIAN_POINT ( 'NONE',  ( -5.207209108562804722, 2.318398865532109276, -15.31249999590322552 ) ) ;
#13708=( BOUNDED_SURFACE ( )  B_SPLINE_SURFACE ( 1, 2, ( 
 ( #10997, #4894, #6467, #12797, #12895, #2083, #12603, #2182, #17101, #18690, #14194, #11395, #595, #18993, #15695, #1985, #11195 ),
 ( #17295, #3584, #5284, #693, #4988, #11095, #17495, #9504, #3394, #17197, #14295, #9406, #15797, #9708, #8287, #15505, #1791 ) ),
 .UNSPECIFIED., .F., .F., .F. ) 
 B_SPLINE_SURFACE_WITH_KNOTS ( ( 2, 2 ),
 ( 3, 2, 2, 2, 2, 2, 2, 2, 3 ),
 ( 0.000000000000000000, 1.000000000000000000 ),
 ( 0.000000000000000000, 0.05000000000000000278, 0.1000000000000000056, 0.1499999999999999944, 0.2000000000000000111, 0.2500000000000000000, 0.2999999999999999889, 0.3499999999999999778, 0.4000000000000000222 ),
 .UNSPECIFIED. ) 
 GEOMETRIC_REPRESENTATION_ITEM ( )  RATIONAL_B_SPLINE_SURFACE ( (
 ( 1.000000000000000000, 0.9876883405951377704, 1.000000000000000000, 0.9876883405951377704, 1.000000000000000000, 0.9876883405951377704, 1.000000000000000000, 0.9876883405951377704, 1.000000000000000000, 0.9876883405951377704, 1.000000000000000000, 0.9876883405951377704, 1.000000000000000000, 0.9876883405951377704, 1.000000000000000000, 0.9876883405951377704, 1.000000000000000000),
 ( 1.000000000000000000, 0.9876883405951377704, 1.000000000000000000, 0.9876883405951377704, 1.000000000000000000, 0.9876883405951377704, 1.000000000000000000, 0.9876883405951377704, 1.000000000000000000, 0.9876883405951377704, 1.000000000000000000, 0.9876883405951377704, 1.000000000000000000, 0.9876883405951377704, 1.000000000000000000, 0.9876883405951377704, 1.000000000000000000) ) ) 
 REPRESENTATION_ITEM ( '' )  SURFACE ( )  );
#13716=CIRCLE ( 'NONE', #14680, 4.200000000000001954 ) ;
#13717=CARTESIAN_POINT ( 'NONE',  ( -0.2590123213420975623, 4.942249507334556924, -8.343749997951613651 ) ) ;
#13723=CARTESIAN_POINT ( 'NONE',  ( 0.7741991708318884946, 4.888101187500000222, -12.34374999795161543 ) ) ;
#13724=CARTESIAN_POINT ( 'NONE',  ( -3.954556930911881096, -2.873153789725797935, -14.84374999795161543 ) ) ;
#13728=EDGE_CURVE ( 'NONE', #4362, #7839, #4999, .T. ) ;
#13735=AXIS2_PLACEMENT_3D ( 'NONE', #6507, #15732, #535 ) ;
#13746=EDGE_CURVE ( 'NONE', #6178, #5524, #12931, .T. ) ;
#13749=AXIS2_PLACEMENT_3D ( 'NONE', #3122, #12531, #9634 ) ;
#13750=PLANE ( 'NONE',  #356 ) ;
#13751=LINE ( 'NONE', #12354, #11924 ) ;
#13812=EDGE_LOOP ( 'NONE', ( #115, #3364, #17969, #6704, #17432, #14134, #15368, #15456, #3015, #4472, #17141, #19724, #12366, #8177, #14892, #16960, #10653 ) ) ;
#13825=CARTESIAN_POINT ( 'NONE',  ( -4.888101187500000222, 0.7741991708318887166, -6.968749997951614539 ) ) ;
#13827=( BOUNDED_SURFACE ( )  B_SPLINE_SURFACE ( 1, 2, ( 
 ( #5295, #3596, #15805, #9814, #15907, #18899, #16205, #10104, #11596, #2093, #17408, #13005, #896, #10011, #16109, #803, #14699 ),
 ( #9717, #14514, #2388, #17697, #988, #3993, #3693, #2189, #8502, #13097, #2478, #6679, #604, #8296, #14607, #8592, #6974 ) ),
 .UNSPECIFIED., .F., .F., .F. ) 
 B_SPLINE_SURFACE_WITH_KNOTS ( ( 2, 2 ),
 ( 3, 2, 2, 2, 2, 2, 2, 2, 3 ),
 ( 0.000000000000000000, 1.000000000000000000 ),
 ( 0.000000000000000000, 0.05000000000000000278, 0.1000000000000000056, 0.1499999999999999944, 0.2000000000000000111, 0.2500000000000000000, 0.2999999999999999889, 0.3499999999999999778, 0.4000000000000000222 ),
 .UNSPECIFIED. ) 
 GEOMETRIC_REPRESENTATION_ITEM ( )  RATIONAL_B_SPLINE_SURFACE ( (
 ( 1.000000000000000000, 0.9876883405951377704, 1.000000000000000000, 0.9876883405951377704, 1.000000000000000000, 0.9876883405951377704, 1.000000000000000000, 0.9876883405951377704, 1.000000000000000000, 0.9876883405951377704, 1.000000000000000000, 0.9876883405951377704, 1.000000000000000000, 0.9876883405951377704, 1.000000000000000000, 0.9876883405951377704, 1.000000000000000000),
 ( 1.000000000000000000, 0.9876883405951377704, 1.000000000000000000, 0.9876883405951377704, 1.000000000000000000, 0.9876883405951377704, 1.000000000000000000, 0.9876883405951377704, 1.000000000000000000, 0.9876883405951377704, 1.000000000000000000, 0.9876883405951377704, 1.000000000000000000, 0.9876883405951377704, 1.000000000000000000, 0.9876883405951377704, 1.000000000000000000) ) ) 
 REPRESENTATION_ITEM ( '' )  SURFACE ( )  );
#13839=CARTESIAN_POINT ( 'NONE',  ( -5.207209108562852684, -2.318398865532001363, -8.000000000000005329 ) ) ;
#13844=CARTESIAN_POINT ( 'NONE',  ( 0.000000000000000000, 0.000000000000000000, -22.00000000000000000 ) ) ;
#13859=ORIENTED_EDGE ( 'NONE', *, *, #12598, .F. ) ;
#13864=ORIENTED_EDGE ( 'NONE', *, *, #10114, .T. ) ;
#13867=CARTESIAN_POINT ( 'NONE',  ( 4.780397808154257078, -1.280903732194453637, -14.34374999795161365 ) ) ;
#13887=FACE_OUTER_BOUND ( 'NONE', #544, .T. ) ;
#13891=CARTESIAN_POINT ( 'NONE',  ( 3.350375938067096548, 4.611396867937201272, -13.00000000000000533 ) ) ;
#13897=LINE ( 'NONE', #1883, #10397 ) ;
#13902=ORIENTED_EDGE ( 'NONE', *, *, #4649, .F. ) ;
#13905=CARTESIAN_POINT ( 'NONE',  ( 9.000000000000001776, 1.102182119232617911E-15, -22.00000000000000000 ) ) ;
#13911=EDGE_CURVE ( 'NONE', #9061, #17079, #11660, .T. ) ;
#13928=CARTESIAN_POINT ( 'NONE',  ( -4.888101187500000222, 0.000000000000000000, -6.468749997951615427 ) ) ;
#13940=CARTESIAN_POINT ( 'NONE',  ( 4.150607464521812062, 2.695436003842704764, -7.968749997951616315 ) ) ;
#13956=ORIENTED_EDGE ( 'NONE', *, *, #14016, .T. ) ;
#13964=CARTESIAN_POINT ( 'NONE',  ( 4.233219804643887585, 2.444050593749991229, -11.84374999795161365 ) ) ;
#13970=AXIS2_PLACEMENT_3D ( 'NONE', #7158, #7059, #2768 ) ;
#13978=DIRECTION ( 'NONE',  ( -0.000000000000000000, -0.000000000000000000, 1.000000000000000000 ) ) ;
#13982=ORIENTED_EDGE ( 'NONE', *, *, #216, .F. ) ;
#13984=CARTESIAN_POINT ( 'NONE',  ( 2.068159791354145849, -5.387740456496247887, -7.812499995903224637 ) ) ;
#13985=CARTESIAN_POINT ( 'NONE',  ( -5.700000000000001066, 0.2987243419133610023, -12.83455515208546238 ) ) ;
#13988=CARTESIAN_POINT ( 'NONE',  ( -3.270778111535288080, 3.632567103900569361, -12.84374999795161543 ) ) ;
#14013=CARTESIAN_POINT ( 'NONE',  ( -4.409619785863906571, 2.246813503491833508, -8.343749997951613651 ) ) ;
#14016=EDGE_CURVE ( 'NONE', #19358, #19556, #13716, .T. ) ;
#14030=CARTESIAN_POINT ( 'NONE',  ( 5.387740456496221242, -2.068159791354220900, -11.81249999590322552 ) ) ;
#14034=CARTESIAN_POINT ( 'NONE',  ( 4.150607464521812062, 2.695436003842704764, -7.968749997951616315 ) ) ;
#14035=CARTESIAN_POINT ( 'NONE',  ( 4.781284448697187273, -1.016293382781444654, -10.84374999795161543 ) ) ;
#14057=VERTEX_POINT ( 'NONE', #12971 ) ;
#14061=VECTOR ( 'NONE', #915, 1000.000000000000000 ) ;
#14076=CARTESIAN_POINT ( 'NONE',  ( -3.814044456245531567, -4.235925505221111997, -11.31249999590322375 ) ) ;
#14077=DIRECTION ( 'NONE',  ( 0.4330127018922130255, -0.7500000000000049960, 0.4999999999999980571 ) ) ;
#14079=CARTESIAN_POINT ( 'NONE',  ( -3.814044456245444081, 4.235925505221192822, -13.31249999590322730 ) ) ;
#14080=ORIENTED_EDGE ( 'NONE', *, *, #17655, .F. ) ;
#14095=CARTESIAN_POINT ( 'NONE',  ( -2.849999999999989431, 4.936344801571308061, -7.312499995903225525 ) ) ;
#14107=CARTESIAN_POINT ( 'NONE',  ( 2.246813503491833508, 4.409619785863906571, -13.34374999795161365 ) ) ;
#14123=ORIENTED_EDGE ( 'NONE', *, *, #13911, .T. ) ;
#14134=ORIENTED_EDGE ( 'NONE', *, *, #12380, .F. ) ;
#14143=CARTESIAN_POINT ( 'NONE',  ( -1.988169868018624609, -4.465502636338009701, -9.468749997951615427 ) ) ;
#14151=ORIENTED_EDGE ( 'NONE', *, *, #6214, .F. ) ;
#14163=CARTESIAN_POINT ( 'NONE',  ( -2.444050593750049849, -4.233219804643852946, -6.843749997951615427 ) ) ;
#14177=CARTESIAN_POINT ( 'NONE',  ( -2.850000000000058265, -4.936344801571268093, -6.000000000000005329 ) ) ;
#14182=CARTESIAN_POINT ( 'NONE',  ( -4.888101187500000222, 0.7741991708318887166, -6.968749997951614539 ) ) ;
#14194=CARTESIAN_POINT ( 'NONE',  ( -3.383411828340740850E-14, -4.888101187500000222, -11.46874999795161543 ) ) ;
#14200=PLANE ( 'NONE',  #4716 ) ;
#14225=CARTESIAN_POINT ( 'NONE',  ( 2.246813503491833508, 4.409619785863906571, -12.96874999795161543 ) ) ;
#14230=ORIENTED_EDGE ( 'NONE', *, *, #631, .F. ) ;
#14232=CARTESIAN_POINT ( 'NONE',  ( -3.846120219227966430, -3.114526743279228072, -11.34374999795161543 ) ) ;
#14246=CARTESIAN_POINT ( 'NONE',  ( 1.773574444220693103, -4.620319390059842490, -6.968749997951614539 ) ) ;
#14266=CARTESIAN_POINT ( 'NONE',  ( -4.942249507334554259, 0.2590123213421660631, -10.34374999795161543 ) ) ;
#14274=ORIENTED_EDGE ( 'NONE', *, *, #5204, .T. ) ;
#14281=EDGE_CURVE ( 'NONE', #1617, #11735, #3365, .T. ) ;
#14295=CARTESIAN_POINT ( 'NONE',  ( -3.945386292505473391E-14, -5.700000000000001066, -11.00000000000000711 ) ) ;
#14298=CARTESIAN_POINT ( 'NONE',  ( -0.3020334839682480288, 5.763142191869157216, -8.812499995903225525 ) ) ;
#14299=ORIENTED_EDGE ( 'NONE', *, *, #5204, .F. ) ;
#14325=CARTESIAN_POINT ( 'NONE',  ( 3.954556930911861112, 2.873153789725825913, -14.46874999795161720 ) ) ;
#14335=CARTESIAN_POINT ( 'NONE',  ( 4.233219804643871598, -2.444050593750019651, -11.84374999795161365 ) ) ;
#14348=CARTESIAN_POINT ( 'NONE',  ( 3.499494075959792116, -3.499494075959840966, -8.968749997951613651 ) ) ;
#14352=ORIENTED_EDGE ( 'NONE', *, *, #16681, .T. ) ;
#14365=ADVANCED_FACE ( 'NONE', ( #12133 ), #13186, .T. ) ;
#14380=CARTESIAN_POINT ( 'NONE',  ( -5.668774803599165857, -0.5958122406255588199, -9.000000000000005329 ) ) ;
#14395=EDGE_CURVE ( 'NONE', #6321, #8931, #7676, .T. ) ;
#14402=CARTESIAN_POINT ( 'NONE',  ( 1.493657965219523875, 5.574407415329157622, -9.812499995903225525 ) ) ;
#14412=CARTESIAN_POINT ( 'NONE',  ( -4.409619785863906571, 2.246813503491833508, -8.343749997951611874 ) ) ;
#14428=ADVANCED_FACE ( 'NONE', ( #15899 ), #13708, .T. ) ;
#14434=CARTESIAN_POINT ( 'NONE',  ( 0.9027913098498565603, 5.700000000000000178, -12.81249999590322552 ) ) ;
#14440=CARTESIAN_POINT ( 'NONE',  ( -0.5958122406255597081, 5.668774803599165857, -15.31249999590322552 ) ) ;
#14447=CARTESIAN_POINT ( 'NONE',  ( -3.954556930911881096, -2.873153789725797935, -14.84374999795161543 ) ) ;
#14449=DIRECTION ( 'NONE',  ( 1.000000000000000000, 0.000000000000000000, 0.000000000000000000 ) ) ;
#14451=CARTESIAN_POINT ( 'NONE',  ( -5.207209108562804722, 2.318398865532109276, -15.31249999590322552 ) ) ;
#14464=CARTESIAN_POINT ( 'NONE',  ( 4.888101187500000222, -3.413342815706642518E-14, -6.843749997951615427 ) ) ;
#14482=CARTESIAN_POINT ( 'NONE',  ( -1.988169868018530906, 4.465502636338051445, -13.84374999795161543 ) ) ;
#14487=CARTESIAN_POINT ( 'NONE',  ( 4.781284448697194378, 1.016293382781411792, -12.46874999795161543 ) ) ;
#14490=CARTESIAN_POINT ( 'NONE',  ( -5.575441324182679459, 1.185096637661293251, -10.00000000000000533 ) ) ;
#14500=CARTESIAN_POINT ( 'NONE',  ( 0.000000000000000000, 0.000000000000000000, -22.00000000000000000 ) ) ;
#14514=CARTESIAN_POINT ( 'NONE',  ( 3.114526743279282694, 3.846120219227923798, -7.343749997951615427 ) ) ;
#14533=CARTESIAN_POINT ( 'NONE',  ( -5.700000000000001954, 6.980486755139915080E-16, 0.000000000000000000 ) ) ;
#14549=CARTESIAN_POINT ( 'NONE',  ( 2.246813503491803310, -4.409619785863921670, -10.34374999795161543 ) ) ;
#14552=CARTESIAN_POINT ( 'NONE',  ( 5.699999999999994849, -0.9027913098498966393, -6.500000000000005329 ) ) ;
#14555=EDGE_LOOP ( 'NONE', ( #10728, #9462 ) ) ;
#14561=CARTESIAN_POINT ( 'NONE',  ( 0.000000000000000000, 0.000000000000000000, -6.000000000000005329 ) ) ;
#14577=CARTESIAN_POINT ( 'NONE',  ( -2.444050593750049849, -4.233219804643852946, -6.468749997951615427 ) ) ;
#14588=CARTESIAN_POINT ( 'NONE',  ( -1.185096637661215091, 5.575441324182695446, -7.000000000000005329 ) ) ;
#14595=( BOUNDED_SURFACE ( )  B_SPLINE_SURFACE ( 1, 2, ( 
 ( #7774, #13984, #6263, #369, #18578, #4876, #15585, #1874, #14076, #6451, #274, #180, #10884, #12388, #16990, #3272, #37 ),
 ( #10836, #3330, #18727, #8016, #12437, #4729, #15541, #15441, #230, #14232, #3226, #5023, #8126, #537, #17041, #11134, #18631 ) ),
 .UNSPECIFIED., .F., .F., .F. ) 
 B_SPLINE_SURFACE_WITH_KNOTS ( ( 2, 2 ),
 ( 3, 2, 2, 2, 2, 2, 2, 2, 3 ),
 ( 0.000000000000000000, 1.000000000000000000 ),
 ( 0.000000000000000000, 0.05000000000000000278, 0.1000000000000000056, 0.1499999999999999944, 0.2000000000000000111, 0.2500000000000000000, 0.2999999999999999889, 0.3499999999999999778, 0.4000000000000000222 ),
 .UNSPECIFIED. ) 
 GEOMETRIC_REPRESENTATION_ITEM ( )  RATIONAL_B_SPLINE_SURFACE ( (
 ( 1.000000000000000000, 0.9876883405951377704, 1.000000000000000000, 0.9876883405951377704, 1.000000000000000000, 0.9876883405951377704, 1.000000000000000000, 0.9876883405951377704, 1.000000000000000000, 0.9876883405951377704, 1.000000000000000000, 0.9876883405951377704, 1.000000000000000000, 0.9876883405951377704, 1.000000000000000000, 0.9876883405951377704, 1.000000000000000000),
 ( 1.000000000000000000, 0.9876883405951377704, 1.000000000000000000, 0.9876883405951377704, 1.000000000000000000, 0.9876883405951377704, 1.000000000000000000, 0.9876883405951377704, 1.000000000000000000, 0.9876883405951377704, 1.000000000000000000, 0.9876883405951377704, 1.000000000000000000, 0.9876883405951377704, 1.000000000000000000, 0.9876883405951377704, 1.000000000000000000) ) ) 
 REPRESENTATION_ITEM ( '' )  SURFACE ( )  );
#14607=CARTESIAN_POINT ( 'NONE',  ( 1.988169868018562880, -4.465502636338038123, -13.84374999795161543 ) ) ;
#14620=PLANE ( 'NONE',  #19544 ) ;
#14631=EDGE_LOOP ( 'NONE', ( #16319, #13128, #9771, #7044, #15711 ) ) ;
#14633=CARTESIAN_POINT ( 'NONE',  ( 3.350375938067096548, 4.611396867937201272, -14.31249999590322552 ) ) ;
#14645=CARTESIAN_POINT ( 'NONE',  ( -2.620002426024580000, -5.142044285764733935, -13.81249999590322552 ) ) ;
#14649=CARTESIAN_POINT ( 'NONE',  ( 5.421022142882364392, -1.761396867937238486, -7.000000000000005329 ) ) ;
#14659=CARTESIAN_POINT ( 'NONE',  ( -3.383411828340740850E-14, -4.888101187500000222, -11.84374999795161365 ) ) ;
#14674=EDGE_CURVE ( 'NONE', #736, #12976, #15764, .T. ) ;
#14676=EDGE_CURVE ( 'NONE', #16711, #4579, #1073, .T. ) ;
#14679=CARTESIAN_POINT ( 'NONE',  ( -5.700000000000001954, 6.980486755139915080E-16, 0.000000000000000000 ) ) ;
#14680=AXIS2_PLACEMENT_3D ( 'NONE', #1156, #2642, #2540 ) ;
#14699=CARTESIAN_POINT ( 'NONE',  ( 0.5958122406255995651, -5.668774803599162304, -15.31249999590322552 ) ) ;
#14700=CARTESIAN_POINT ( 'NONE',  ( 4.465502636338039011, 1.988169868018562436, -8.468749997951615427 ) ) ;
#14705=( BOUNDED_CURVE ( )  B_SPLINE_CURVE ( 2, ( #15934, #3725, #4017, #8616, #3820, #16323, #13225, #6809, #2603, #14821, #5220, #14434, #9845, #10129, #14633, #2317, #732 ),
 .UNSPECIFIED., .F., .F. ) 
 B_SPLINE_CURVE_WITH_KNOTS ( ( 3, 2, 2, 2, 2, 2, 2, 2, 3 ),
 ( 0.000000000000000000, 0.05000000000000000971, 0.1000000000000000194, 0.1499999999999999944, 0.2000000000000000389, 0.2500000000000000000, 0.2999999999999999889, 0.3499999999999999223, 0.4000000000000000777 ),
 .UNSPECIFIED. ) 
 CURVE ( )  GEOMETRIC_REPRESENTATION_ITEM ( )  RATIONAL_B_SPLINE_CURVE ( ( 1.000000000000000000, 0.9876883405951377704, 1.000000000000000000, 0.9876883405951377704, 1.000000000000000000, 0.9876883405951377704, 1.000000000000000000, 0.9876883405951377704, 1.000000000000000000, 0.9876883405951377704, 1.000000000000000000, 0.9876883405951377704, 1.000000000000000000, 0.9876883405951377704, 1.000000000000000000, 0.9876883405951377704, 1.000000000000000000 ) ) 
 REPRESENTATION_ITEM ( '' )  );
#14708=COLOUR_RGB ( '', 0.31764706, 0.68627451, 0.89019608) ;
#14718=CARTESIAN_POINT ( 'NONE',  ( 3.632567103900546712, 3.270778111535313837, -7.843749997951614539 ) ) ;
#14732=ORIENTED_EDGE ( 'NONE', *, *, #17045, .F. ) ;
#14748=DIRECTION ( 'NONE',  ( -0.1045284632676491549, 0.9945218953682738450, 0.000000000000000000 ) ) ;
#14751=CARTESIAN_POINT ( 'NONE',  ( -3.383411828340740850E-14, -4.888101187500000222, -11.46874999795161543 ) ) ;
#14756=CIRCLE ( 'NONE', #19517, 9.000000000000000000 ) ;
#14757=DIRECTION ( 'NONE',  ( 0.000000000000000000, 0.000000000000000000, -1.000000000000000000 ) ) ;
#14795=CARTESIAN_POINT ( 'NONE',  ( 5.700000000000002842, 9.001153973733047589E-16, -18.00000000000000355 ) ) ;
#14800=CARTESIAN_POINT ( 'NONE',  ( 0.5109457054261454800, -4.861323657744410554, -14.46874999795161720 ) ) ;
#14801=CARTESIAN_POINT ( 'NONE',  ( -4.233219804643904460, -2.444050593749961031, -11.84374999795161365 ) ) ;
#14821=CARTESIAN_POINT ( 'NONE',  ( -0.9027913098498572264, 5.700000000000000178, -11.81249999590322552 ) ) ;
#14824=CARTESIAN_POINT ( 'NONE',  ( 2.620002426024544029, 5.142044285764751699, -12.50000000000000533 ) ) ;
#14826=CARTESIAN_POINT ( 'NONE',  ( -4.233219804643904460, -2.444050593749961031, -11.46874999795161543 ) ) ;
#14836=CARTESIAN_POINT ( 'NONE',  ( 3.631840208645826795, 4.484949146646356688, -6.500000000000005329 ) ) ;
#14844=ADVANCED_FACE ( 'NONE', ( #16363 ), #6158, .T. ) ;
#14856=EDGE_CURVE ( 'NONE', #488, #6321, #16128, .T. ) ;
#14864=CARTESIAN_POINT ( 'NONE',  ( -3.632567103900569361, -3.270778111535287191, -7.468749997951615427 ) ) ;
#14866=PLANE ( 'NONE',  #9363 ) ;
#14888=EDGE_CURVE ( 'NONE', #17046, #1346, #7028, .T. ) ;
#14892=ORIENTED_EDGE ( 'NONE', *, *, #16236, .F. ) ;
#14893=DIRECTION ( 'NONE',  ( 0.000000000000000000, 0.000000000000000000, 1.000000000000000000 ) ) ;
#14925=CARTESIAN_POINT ( 'NONE',  ( -0.5109457054262123155, -4.861323657744403448, -8.468749997951615427 ) ) ;
#14931=CARTESIAN_POINT ( 'NONE',  ( -1.510506337161893642, -4.648860486681943627, -12.84374999795161543 ) ) ;
#14934=CARTESIAN_POINT ( 'NONE',  ( -2.444050593749990341, 4.233219804643887585, -6.656249997951614539 ) ) ;
#14943=CARTESIAN_POINT ( 'NONE',  ( 2.246813503491803310, -4.409619785863921670, -9.968749997951617203 ) ) ;
#14962=CARTESIAN_POINT ( 'NONE',  ( 1.988169868018593300, 4.465502636338023912, -9.468749997951615427 ) ) ;
#14964=CARTESIAN_POINT ( 'NONE',  ( -4.861323657744403448, 0.5109457054262118714, -13.46874999795161543 ) ) ;
#14980=ADVANCED_FACE ( 'NONE', ( #9658 ), #15655, .T. ) ;
#14982=CARTESIAN_POINT ( 'NONE',  ( -2.620002426024580000, -5.142044285764733935, -13.81249999590322730 ) ) ;
#14985=ORIENTED_EDGE ( 'NONE', *, *, #9164, .F. ) ;
#14992=DIRECTION ( 'NONE',  ( -0.000000000000000000, -0.000000000000000000, 1.000000000000000000 ) ) ;
#14993=PRODUCT_DEFINITION_FORMATION_WITH_SPECIFIED_SOURCE ( 'ANY', '', #15935, .NOT_KNOWN. ) ;
#14999=CARTESIAN_POINT ( 'NONE',  ( -4.465502636338051445, -1.988169868018530462, -8.468749997951615427 ) ) ;
#15015=VERTEX_POINT ( 'NONE', #6625 ) ;
#15020=CARTESIAN_POINT ( 'NONE',  ( -1.773574444220725521, 4.620319390059830056, -7.343749997951615427 ) ) ;
#15026=ORIENTED_EDGE ( 'NONE', *, *, #15427, .F. ) ;
#15032=CARTESIAN_POINT ( 'NONE',  ( 4.620319390059829168, 1.773574444220725299, -12.34374999795161543 ) ) ;
#15037=ORIENTED_EDGE ( 'NONE', *, *, #838, .F. ) ;
#15053=CARTESIAN_POINT ( 'NONE',  ( -9.000000000000001776, 1.102182119232617911E-15, 0.000000000000000000 ) ) ;
#15057=CARTESIAN_POINT ( 'NONE',  ( 5.668774803599163192, 0.5958122406255991210, -9.000000000000005329 ) ) ;
#15063=CARTESIAN_POINT ( 'NONE',  ( 5.668774803599156975, -0.5958122406256377568, -13.00000000000000533 ) ) ;
#15070=CARTESIAN_POINT ( 'NONE',  ( -2.068159791354184041, 5.387740456496233676, -7.812499995903224637 ) ) ;
#15093=CARTESIAN_POINT ( 'NONE',  ( -5.700000000000001066, 1.090170143537592985E-15, -9.332722423957234170 ) ) ;
#15100=CARTESIAN_POINT ( 'NONE',  ( -4.620319390059805187, 1.773574444220789914, -10.96874999795161720 ) ) ;
#15115=( BOUNDED_SURFACE ( )  B_SPLINE_SURFACE ( 1, 2, ( 
 ( #10888, #14182, #16994, #278, #6556, #9289, #10985, #1877, #17186, #18680, #11082, #18778, #9586, #184, #8072, #6174, #3278 ),
 ( #5070, #16898, #7971, #11183, #373, #2072, #9695, #6455, #1779, #12295, #7870, #3179, #7778, #12588, #13891, #6267, #12487 ) ),
 .UNSPECIFIED., .F., .F., .F. ) 
 B_SPLINE_SURFACE_WITH_KNOTS ( ( 2, 2 ),
 ( 3, 2, 2, 2, 2, 2, 2, 2, 3 ),
 ( 0.000000000000000000, 1.000000000000000000 ),
 ( 0.000000000000000000, 0.05000000000000000278, 0.1000000000000000056, 0.1499999999999999944, 0.2000000000000000111, 0.2500000000000000000, 0.2999999999999999889, 0.3499999999999999778, 0.4000000000000000222 ),
 .UNSPECIFIED. ) 
 GEOMETRIC_REPRESENTATION_ITEM ( )  RATIONAL_B_SPLINE_SURFACE ( (
 ( 1.000000000000000000, 0.9876883405951377704, 1.000000000000000000, 0.9876883405951377704, 1.000000000000000000, 0.9876883405951377704, 1.000000000000000000, 0.9876883405951377704, 1.000000000000000000, 0.9876883405951377704, 1.000000000000000000, 0.9876883405951377704, 1.000000000000000000, 0.9876883405951377704, 1.000000000000000000, 0.9876883405951377704, 1.000000000000000000),
 ( 1.000000000000000000, 0.9876883405951377704, 1.000000000000000000, 0.9876883405951377704, 1.000000000000000000, 0.9876883405951377704, 1.000000000000000000, 0.9876883405951377704, 1.000000000000000000, 0.9876883405951377704, 1.000000000000000000, 0.9876883405951377704, 1.000000000000000000, 0.9876883405951377704, 1.000000000000000000, 0.9876883405951377704, 1.000000000000000000) ) ) 
 REPRESENTATION_ITEM ( '' )  SURFACE ( )  );
#15122=CARTESIAN_POINT ( 'NONE',  ( -4.780397808154247308, 1.280903732194486722, -14.34374999795161365 ) ) ;
#15131=CARTESIAN_POINT ( 'NONE',  ( 1.988169868018593300, 4.465502636338023912, -9.843749997951615427 ) ) ;
#15142=CARTESIAN_POINT ( 'NONE',  ( 0.000000000000000000, 0.000000000000000000, -6.000000000000005329 ) ) ;
#15147=AXIS2_PLACEMENT_3D ( 'NONE', #8540, #18845, #14449 ) ;
#15149=ORIENTED_EDGE ( 'NONE', *, *, #9471, .F. ) ;
#15159=DIRECTION ( 'NONE',  ( 1.000000000000000000, 0.000000000000000000, 0.000000000000000000 ) ) ;
#15163=CARTESIAN_POINT ( 'NONE',  ( 0.3020334839682081163, -5.763142191869158992, -8.812499995903225525 ) ) ;
#15166=CARTESIAN_POINT ( 'NONE',  ( -2.444050593750049849, -4.233219804643852946, -6.468749997951615427 ) ) ;
#15167=CARTESIAN_POINT ( 'NONE',  ( 4.484949146646379781, 3.631840208645794821, -11.81249999590322552 ) ) ;
#15176=VECTOR ( 'NONE', #7031, 1000.000000000000000 ) ;
#15181=CARTESIAN_POINT ( 'NONE',  ( -3.350375938067128967, -4.611396867937178179, -14.31249999590322552 ) ) ;
#15196=ORIENTED_EDGE ( 'NONE', *, *, #19203, .T. ) ;
#15198=CARTESIAN_POINT ( 'NONE',  ( -0.5109457054261112852, 4.861323657744413218, -14.46874999795161720 ) ) ;
#15199=APPLICATION_CONTEXT ( 'automotive_design' ) ;
#15212=CARTESIAN_POINT ( 'NONE',  ( 3.270778111535314281, -3.632567103900546712, -12.84374999795161543 ) ) ;
#15224=CARTESIAN_POINT ( 'NONE',  ( 4.620319390059829168, 1.773574444220725743, -12.34374999795161543 ) ) ;
#15231=CARTESIAN_POINT ( 'NONE',  ( -4.648860486681953397, 1.510506337161861445, -7.468749997951615427 ) ) ;
#15233=( BOUNDED_CURVE ( )  B_SPLINE_CURVE ( 2, ( #3151, #11963, #7438, #15163, #16471, #50, #7749, #16667, #2948, #18267, #15367, #4552, #3049, #154, #1654 ),
 .UNSPECIFIED., .F., .F. ) 
 B_SPLINE_CURVE_WITH_KNOTS ( ( 3, 2, 2, 2, 2, 2, 2, 3 ),
 ( 0.000000000000000000, 0.05000000000000000278, 0.1000000000000000056, 0.1499999999999999944, 0.2000000000000000111, 0.2500000000000000000, 0.2999999999999999889, 0.3333180920165860761 ),
 .UNSPECIFIED. ) 
 CURVE ( )  GEOMETRIC_REPRESENTATION_ITEM ( )  RATIONAL_B_SPLINE_CURVE ( ( 1.000000000000000000, 0.9876883405951377704, 1.000000000000000000, 0.9876883405951377704, 1.000000000000000000, 0.9876883405951377704, 1.000000000000000000, 0.9876883405951377704, 1.000000000000000000, 0.9876883405951377704, 1.000000000000000000, 0.9876883405951377704, 1.000000000000000000, 0.9917959799814386468, 0.9945256517182510247 ) ) 
 REPRESENTATION_ITEM ( '' )  );
#15237=CARTESIAN_POINT ( 'NONE',  ( -2.246813503491833508, 4.409619785863906571, -9.968749997951615427 ) ) ;
#15249=EDGE_CURVE ( 'NONE', #17369, #6321, #19331, .T. ) ;
#15263=CARTESIAN_POINT ( 'NONE',  ( 3.270778111535314281, -3.632567103900546712, -12.46874999795161543 ) ) ;
#15265=CARTESIAN_POINT ( 'NONE',  ( 4.781284448697194378, 1.016293382781411792, -12.46874999795161543 ) ) ;
#15268=CARTESIAN_POINT ( 'NONE',  ( -2.068159791354183596, 5.387740456496233676, -6.500000000000005329 ) ) ;
#15274=CARTESIAN_POINT ( 'NONE',  ( 3.270778111535338262, 3.632567103900524064, -10.84374999795161543 ) ) ;
#15299=CARTESIAN_POINT ( 'NONE',  ( 2.246813503491833508, 4.409619785863906571, -13.34374999795161365 ) ) ;
#15302=CARTESIAN_POINT ( 'NONE',  ( 0.000000000000000000, 0.000000000000000000, 0.000000000000000000 ) ) ;
#15317=DIRECTION ( 'NONE',  ( -0.000000000000000000, -0.000000000000000000, 1.000000000000000000 ) ) ;
#15342=PLANE ( 'NONE',  #1816 ) ;
#15346=PRESENTATION_STYLE_ASSIGNMENT (( #12142 ) ) ;
#15351=CARTESIAN_POINT ( 'NONE',  ( 5.021782490506621954, -2.235841616153703360, -14.11718749948790830 ) ) ;
#15367=CARTESIAN_POINT ( 'NONE',  ( -4.936344801571327601, -2.849999999999954792, -12.31249999590322552 ) ) ;
#15368=ORIENTED_EDGE ( 'NONE', *, *, #12019, .T. ) ;
#15393=CARTESIAN_POINT ( 'NONE',  ( -1.280903732194386802, 4.780397808154273065, -14.34374999795161365 ) ) ;
#15418=CARTESIAN_POINT ( 'NONE',  ( -4.648860486681953397, 1.510506337161861445, -7.843749997951614539 ) ) ;
#15427=EDGE_CURVE ( 'NONE', #768, #5986, #12431, .T. ) ;
#15428=CARTESIAN_POINT ( 'NONE',  ( -2.873153789725825469, 3.954556930911862000, -9.468749997951615427 ) ) ;
#15441=CARTESIAN_POINT ( 'NONE',  ( -2.695436003842760275, -4.150607464521772094, -10.34374999795161543 ) ) ;
#15448=DIRECTION ( 'NONE',  ( 0.000000000000000000, 0.000000000000000000, -1.000000000000000000 ) ) ;
#15456=ORIENTED_EDGE ( 'NONE', *, *, #12016, .T. ) ;
#15469=DIRECTION ( 'NONE',  ( 0.000000000000000000, 0.000000000000000000, -1.000000000000000000 ) ) ;
#15470=CARTESIAN_POINT ( 'NONE',  ( -1.016293382781411569, 4.781284448697194378, -7.843749997951614539 ) ) ;
#15472=( BOUNDED_SURFACE ( )  B_SPLINE_SURFACE ( 1, 2, ( 
 ( #19325, #17935, #745, #7201, #6919, #8537, #17832, #16436, #6822, #4126, #19425, #9953, #5709, #14645, #5332, #10140, #11826 ),
 ( #13134, #11445, #19230, #10238, #16332, #17545, #2330, #14549, #842, #5424, #2713, #16044, #11536, #8625, #11730, #3931, #14447 ) ),
 .UNSPECIFIED., .F., .F., .F. ) 
 B_SPLINE_SURFACE_WITH_KNOTS ( ( 2, 2 ),
 ( 3, 2, 2, 2, 2, 2, 2, 2, 3 ),
 ( 0.000000000000000000, 1.000000000000000000 ),
 ( 0.000000000000000000, 0.05000000000000000278, 0.1000000000000000056, 0.1499999999999999944, 0.2000000000000000111, 0.2500000000000000000, 0.2999999999999999889, 0.3499999999999999778, 0.4000000000000000222 ),
 .UNSPECIFIED. ) 
 GEOMETRIC_REPRESENTATION_ITEM ( )  RATIONAL_B_SPLINE_SURFACE ( (
 ( 1.000000000000000000, 0.9876883405951377704, 1.000000000000000000, 0.9876883405951377704, 1.000000000000000000, 0.9876883405951377704, 1.000000000000000000, 0.9876883405951377704, 1.000000000000000000, 0.9876883405951377704, 1.000000000000000000, 0.9876883405951377704, 1.000000000000000000, 0.9876883405951377704, 1.000000000000000000, 0.9876883405951377704, 1.000000000000000000),
 ( 1.000000000000000000, 0.9876883405951377704, 1.000000000000000000, 0.9876883405951377704, 1.000000000000000000, 0.9876883405951377704, 1.000000000000000000, 0.9876883405951377704, 1.000000000000000000, 0.9876883405951377704, 1.000000000000000000, 0.9876883405951377704, 1.000000000000000000, 0.9876883405951377704, 1.000000000000000000, 0.9876883405951377704, 1.000000000000000000) ) ) 
 REPRESENTATION_ITEM ( '' )  SURFACE ( )  );
#15482=CARTESIAN_POINT ( 'NONE',  ( 0.000000000000000000, 0.000000000000000000, -6.000000000000005329 ) ) ;
#15505=CARTESIAN_POINT ( 'NONE',  ( -4.080749450109677490, -4.080749450109621534, -13.50000000000000533 ) ) ;
#15511=ORIENTED_EDGE ( 'NONE', *, *, #7498, .F. ) ;
#15518=EDGE_CURVE ( 'NONE', #13685, #9061, #16307, .T. ) ;
#15541=CARTESIAN_POINT ( 'NONE',  ( -1.988169868018624609, -4.465502636338009701, -9.843749997951615427 ) ) ;
#15543=CARTESIAN_POINT ( 'NONE',  ( 2.444050593750020095, 4.233219804643871598, -6.468749997951615427 ) ) ;
#15545=FACE_OUTER_BOUND ( 'NONE', #18244, .T. ) ;
#15550=CARTESIAN_POINT ( 'NONE',  ( -5.207209108562804722, 2.318398865532109276, -14.00000000000000533 ) ) ;
#15567=ORIENTED_EDGE ( 'NONE', *, *, #11649, .F. ) ;
#15579=EDGE_CURVE ( 'NONE', #3194, #4661, #15828, .T. ) ;
#15583=B_SPLINE_CURVE_WITH_KNOTS ( 'NONE', 1,
 ( #17521, #2496 ),
 .UNSPECIFIED., .F., .F.,
 ( 2, 2 ),
 ( 0.000000000000000000, 1.000000000000000000 ),
 .UNSPECIFIED. ) ;
#15585=CARTESIAN_POINT ( 'NONE',  ( -2.318398865532109721, -5.207209108562803834, -10.31249999590322552 ) ) ;
#15608=DIRECTION ( 'NONE',  ( 0.000000000000000000, -0.000000000000000000, 1.000000000000000000 ) ) ;
#15615=CARTESIAN_POINT ( 'NONE',  ( 1.510506337161861223, 4.648860486681953397, -12.84374999795161543 ) ) ;
#15619=VECTOR ( 'NONE', #4461, 1000.000000000000000 ) ;
#15620=ORIENTED_EDGE ( 'NONE', *, *, #17053, .F. ) ;
#15621=EDGE_CURVE ( 'NONE', #768, #5267, #5409, .T. ) ;
#15624=LINE ( 'NONE', #12721, #700 ) ;
#15638=CARTESIAN_POINT ( 'NONE',  ( -5.574407415329178939, -1.493657965219446160, -8.500000000000005329 ) ) ;
#15639=CARTESIAN_POINT ( 'NONE',  ( 3.114526743279282694, 3.846120219227923798, -6.968749997951614539 ) ) ;
#15655=CYLINDRICAL_SURFACE ( 'NONE', #11328, 5.700000000000001954 ) ;
#15665=( GEOMETRIC_REPRESENTATION_CONTEXT ( 3 ) GLOBAL_UNCERTAINTY_ASSIGNED_CONTEXT ( ( #10198 ) ) GLOBAL_UNIT_ASSIGNED_CONTEXT ( ( #7311, #4238, #11938 ) ) REPRESENTATION_CONTEXT ( 'NONE', 'WORKASPACE' ) );
#15667=CARTESIAN_POINT ( 'NONE',  ( -0.5109457054261112852, 4.861323657744413218, -14.84374999795161543 ) ) ;
#15672=CARTESIAN_POINT ( 'NONE',  ( -5.294050593750000644, 0.000000000000000000, -6.234374998975811266 ) ) ;
#15682=EDGE_CURVE ( 'NONE', #8042, #19358, #17327, .T. ) ;
#15684=CARTESIAN_POINT ( 'NONE',  ( -2.695436003842674566, 4.150607464521828938, -13.34374999795161365 ) ) ;
#15695=CARTESIAN_POINT ( 'NONE',  ( -2.873153789725852558, -3.954556930911842016, -13.46874999795161543 ) ) ;
#15698=FILL_AREA_STYLE ('',( #18499 ) ) ;
#15706=DIRECTION ( 'NONE',  ( 1.000000000000000000, 0.000000000000000000, 0.000000000000000000 ) ) ;
#15711=ORIENTED_EDGE ( 'NONE', *, *, #18807, .T. ) ;
#15724=CARTESIAN_POINT ( 'NONE',  ( -1.493657965219446160, 5.574407415329178939, -14.81249999590322375 ) ) ;
#15730=CARTESIAN_POINT ( 'NONE',  ( 0.000000000000000000, 0.000000000000000000, -6.000000000000005329 ) ) ;
#15732=DIRECTION ( 'NONE',  ( -0.000000000000000000, -0.000000000000000000, 1.000000000000000000 ) ) ;
#15739=CARTESIAN_POINT ( 'NONE',  ( 2.444050593750020095, 4.233219804643871598, -6.843749997951615427 ) ) ;
#15748=CARTESIAN_POINT ( 'NONE',  ( -4.465502636338010589, 1.988169868018623720, -14.46874999795161720 ) ) ;
#15749=CARTESIAN_POINT ( 'NONE',  ( -4.781284448697201483, -1.016293382781378485, -12.46874999795161543 ) ) ;
#15763=VERTEX_POINT ( 'NONE', #1206 ) ;
#15764=( BOUNDED_CURVE ( )  B_SPLINE_CURVE ( 2, ( #10487, #3066, #169, #2765, #6161, #7458, #7354, #19770, #1474, #12280, #13578, #8881, #18378, #14982, #15181, #4377, #4670 ),
 .UNSPECIFIED., .F., .F. ) 
 B_SPLINE_CURVE_WITH_KNOTS ( ( 3, 2, 2, 2, 2, 2, 2, 2, 3 ),
 ( 0.000000000000000000, 0.05000000000000000971, 0.1000000000000000194, 0.1499999999999999944, 0.2000000000000000389, 0.2500000000000000000, 0.2999999999999999889, 0.3499999999999999223, 0.4000000000000000777 ),
 .UNSPECIFIED. ) 
 CURVE ( )  GEOMETRIC_REPRESENTATION_ITEM ( )  RATIONAL_B_SPLINE_CURVE ( ( 1.000000000000000000, 0.9876883405951377704, 1.000000000000000000, 0.9876883405951377704, 1.000000000000000000, 0.9876883405951377704, 1.000000000000000000, 0.9876883405951377704, 1.000000000000000000, 0.9876883405951377704, 1.000000000000000000, 0.9876883405951377704, 1.000000000000000000, 0.9876883405951377704, 1.000000000000000000, 0.9876883405951377704, 1.000000000000000000 ) ) 
 REPRESENTATION_ITEM ( '' )  );
#15771=CARTESIAN_POINT ( 'NONE',  ( -1.280903732194386802, 4.780397808154273065, -14.34374999795161543 ) ) ;
#15776=( GEOMETRIC_REPRESENTATION_CONTEXT ( 3 ) GLOBAL_UNCERTAINTY_ASSIGNED_CONTEXT ( ( #16204 ) ) GLOBAL_UNIT_ASSIGNED_CONTEXT ( ( #6673, #8086, #7986 ) ) REPRESENTATION_CONTEXT ( 'NONE', 'WORKASPACE' ) );
#15783=CARTESIAN_POINT ( 'NONE',  ( -2.318398865532001363, 5.207209108562852684, -13.00000000000000533 ) ) ;
#15785=EDGE_CURVE ( 'NONE', #4579, #5395, #8704, .T. ) ;
#15786=CARTESIAN_POINT ( 'NONE',  ( -3.143139765844555900, 4.840010801796527318, -13.81249999590322552 ) ) ;
#15791=ORIENTED_EDGE ( 'NONE', *, *, #1103, .T. ) ;
#15797=CARTESIAN_POINT ( 'NONE',  ( -1.761396867937238042, -5.421022142882365280, -12.00000000000000533 ) ) ;
#15805=CARTESIAN_POINT ( 'NONE',  ( 4.235925505221166176, 3.814044456245473835, -8.312499995903225525 ) ) ;
#15808=ORIENTED_EDGE ( 'NONE', *, *, #7498, .T. ) ;
#15817=CYLINDRICAL_SURFACE ( 'NONE', #9474, 9.000000000000001776 ) ;
#15828=LINE ( 'NONE', #11225, #16619 ) ;
#15838=CARTESIAN_POINT ( 'NONE',  ( 4.942249507334556036, -0.2590123213421313686, -10.34374999795161543 ) ) ;
#15843=ORIENTED_EDGE ( 'NONE', *, *, #2322, .F. ) ;
#15844=CARTESIAN_POINT ( 'NONE',  ( -4.611396867937224364, -3.350375938067065906, -14.00000000000000533 ) ) ;
#15847=CARTESIAN_POINT ( 'NONE',  ( -2.695436003842760719, -4.150607464521772094, -9.968749997951615427 ) ) ;
#15851=CARTESIAN_POINT ( 'NONE',  ( 4.648860486681943627, -1.510506337161893864, -7.468749997951615427 ) ) ;
#15854=VERTEX_POINT ( 'NONE', #14095 ) ;
#15855=CARTESIAN_POINT ( 'NONE',  ( 2.647025296875021638, 4.584782303107579615, -6.234374998975811266 ) ) ;
#15862=ORIENTED_EDGE ( 'NONE', *, *, #4183, .F. ) ;
#15874=( BOUNDED_CURVE ( )  B_SPLINE_CURVE ( 2, ( #19197, #16119, #995, #7072, #2394, #5303, #2680, #2582, #8509 ),
 .UNSPECIFIED., .F., .F. ) 
 B_SPLINE_CURVE_WITH_KNOTS ( ( 3, 2, 2, 2, 3 ),
 ( 0.000000000000000000, 0.04999999999999999584, 0.09999999999999999167, 0.1499999999999999944, 0.1666819079834116757 ),
 .UNSPECIFIED. ) 
 CURVE ( )  GEOMETRIC_REPRESENTATION_ITEM ( )  RATIONAL_B_SPLINE_CURVE ( ( 1.000000000000000000, 0.9876883405951377704, 1.000000000000000000, 0.9876883405951377704, 1.000000000000000000, 0.9876883405951377704, 1.000000000000000000, 0.9958923606136996787, 0.9945256517182512468 ) ) 
 REPRESENTATION_ITEM ( '' )  );
#15885=CARTESIAN_POINT ( 'NONE',  ( -4.936344801571268093, 2.850000000000057820, -11.00000000000000711 ) ) ;
#15895=EDGE_CURVE ( 'NONE', #5399, #12952, #12410, .T. ) ;
#15899=FACE_OUTER_BOUND ( 'NONE', #1147, .T. ) ;
#15907=CARTESIAN_POINT ( 'NONE',  ( 5.207209108562838473, 2.318398865532038666, -9.312499995903225525 ) ) ;
#15912=CARTESIAN_POINT ( 'NONE',  ( -4.888101187500000222, 0.000000000000000000, -6.843749997951615427 ) ) ;
#15918=CARTESIAN_POINT ( 'NONE',  ( 2.444050593750020095, 4.233219804643871598, -6.468749997951615427 ) ) ;
#15922=LINE ( 'NONE', #9930, #17059 ) ;
#15931=LINE ( 'NONE', #17529, #9512 ) ;
#15934=CARTESIAN_POINT ( 'NONE',  ( -5.700000000000001066, 0.000000000000000000, -7.312499995903225525 ) ) ;
#15935=PRODUCT ( 'DRIVER', 'DRIVER', '', ( #4655 ) ) ;
#15938=CARTESIAN_POINT ( 'NONE',  ( 1.280903732194421663, -4.780397808154265960, -14.34374999795161365 ) ) ;
#15975=CARTESIAN_POINT ( 'NONE',  ( 4.233219804643887585, 2.444050593749990785, -11.46874999795161543 ) ) ;
#15988=EDGE_CURVE ( 'NONE', #15854, #4661, #8975, .T. ) ;
#16024=DIRECTION ( 'NONE',  ( -0.000000000000000000, -0.000000000000000000, 1.000000000000000000 ) ) ;
#16044=CARTESIAN_POINT ( 'NONE',  ( -0.7741991708319226895, -4.888101187499994893, -12.34374999795161543 ) ) ;
#16048=CARTESIAN_POINT ( 'NONE',  ( -2.873153789725852558, -3.954556930911842016, -13.46874999795161543 ) ) ;
#16063=CARTESIAN_POINT ( 'NONE',  ( -0.5958122406255597081, 5.668774803599165857, -14.00000000000000533 ) ) ;
#16064=EDGE_CURVE ( 'NONE', #12845, #5267, #15233, .T. ) ;
#16073=CLOSED_SHELL ( 'NONE', ( #14980, #18184, #2196, #10927, #17393, #6912, #5873, #11431, #16758, #12359, #6104, #8094, #10057, #9227, #19361, #3470, #5041, #18372, #4922, #18712, #8063, #2695, #14365, #4016, #17929, #16180, #10317, #4490, #16811, #11849, #9373, #14428, #13474, #476, #2711, #5300, #2754, #8223, #3463, #10489, #7287, #12969, #14844, #5030 ) ) ;
#16084=CARTESIAN_POINT ( 'NONE',  ( -4.780397808154273953, -1.280903732194386579, -8.968749997951611874 ) ) ;
#16109=CARTESIAN_POINT ( 'NONE',  ( 2.318398865532038666, -5.207209108562836697, -14.31249999590322552 ) ) ;
#16115=CARTESIAN_POINT ( 'NONE',  ( -5.699999999999999289, 0.9027913098498568933, -7.812499995903224637 ) ) ;
#16118=( BOUNDED_SURFACE ( )  B_SPLINE_SURFACE ( 1, 2, ( 
 ( #2544, #11566, #5361, #17477, #12975, #17378, #13169, #1061, #5158, #9888, #15975, #9980, #14487, #19067, #868, #8764, #9161 ),
 ( #5743, #15268, #13267, #1256, #16570, #2746, #4158, #16366, #19357, #1458, #6043, #5650, #4456, #13560, #15063, #18170, #1358 ) ),
 .UNSPECIFIED., .F., .F., .F. ) 
 B_SPLINE_SURFACE_WITH_KNOTS ( ( 2, 2 ),
 ( 3, 2, 2, 2, 2, 2, 2, 2, 3 ),
 ( 0.000000000000000000, 1.000000000000000000 ),
 ( 0.000000000000000000, 0.05000000000000000278, 0.1000000000000000056, 0.1499999999999999944, 0.2000000000000000111, 0.2500000000000000000, 0.2999999999999999889, 0.3499999999999999778, 0.4000000000000000222 ),
 .UNSPECIFIED. ) 
 GEOMETRIC_REPRESENTATION_ITEM ( )  RATIONAL_B_SPLINE_SURFACE ( (
 ( 1.000000000000000000, 0.9876883405951377704, 1.000000000000000000, 0.9876883405951377704, 1.000000000000000000, 0.9876883405951377704, 1.000000000000000000, 0.9876883405951377704, 1.000000000000000000, 0.9876883405951377704, 1.000000000000000000, 0.9876883405951377704, 1.000000000000000000, 0.9876883405951377704, 1.000000000000000000, 0.9876883405951377704, 1.000000000000000000),
 ( 1.000000000000000000, 0.9876883405951377704, 1.000000000000000000, 0.9876883405951377704, 1.000000000000000000, 0.9876883405951377704, 1.000000000000000000, 0.9876883405951377704, 1.000000000000000000, 0.9876883405951377704, 1.000000000000000000, 0.9876883405951377704, 1.000000000000000000, 0.9876883405951377704, 1.000000000000000000, 0.9876883405951377704, 1.000000000000000000) ) ) 
 REPRESENTATION_ITEM ( '' )  SURFACE ( )  );
#16119=CARTESIAN_POINT ( 'NONE',  ( 3.631840208645826795, 4.484949146646356688, -7.812499995903224637 ) ) ;
#16128=CIRCLE ( 'NONE', #1422, 5.700000000000001954 ) ;
#16135=DIRECTION ( 'NONE',  ( 0.000000000000000000, 0.000000000000000000, -1.000000000000000000 ) ) ;
#16169=EDGE_LOOP ( 'NONE', ( #446, #15567 ) ) ;
#16171=CARTESIAN_POINT ( 'NONE',  ( 0.000000000000000000, 5.700000000000001954, -6.000000000000005329 ) ) ;
#16177=CARTESIAN_POINT ( 'NONE',  ( -2.695436003842674566, 4.150607464521828938, -13.34374999795161365 ) ) ;
#16180=ADVANCED_FACE ( 'NONE', ( #13145 ), #8039, .T. ) ;
#16181=ORIENTED_EDGE ( 'NONE', *, *, #14856, .F. ) ;
#16184=CARTESIAN_POINT ( 'NONE',  ( -2.444050593750049849, -4.233219804643852946, -6.468749997951615427 ) ) ;
#16204=UNCERTAINTY_MEASURE_WITH_UNIT (LENGTH_MEASURE( 1.000000000000000082E-05 ), #6673, 'distance_accuracy_value', 'NONE');
#16205=CARTESIAN_POINT ( 'NONE',  ( 5.668774803599163192, 0.5958122406255991210, -10.31249999590322552 ) ) ;
#16208=CARTESIAN_POINT ( 'NONE',  ( -1.761396867937200739, 5.421022142882375938, -11.31249999590322375 ) ) ;
#16225=ORIENTED_EDGE ( 'NONE', *, *, #18082, .T. ) ;
#16231=CARTESIAN_POINT ( 'NONE',  ( 2.444050593749960587, -4.233219804643904460, -6.843749997951615427 ) ) ;
#16236=EDGE_CURVE ( 'NONE', #9061, #488, #7638, .T. ) ;
#16242=DIRECTION ( 'NONE',  ( 0.8660254037844330455, -0.5000000000000098810, 0.000000000000000000 ) ) ;
#16269=CARTESIAN_POINT ( 'NONE',  ( -4.150607464521828938, -2.695436003842674566, -8.343749997951611874 ) ) ;
#16281=CARTESIAN_POINT ( 'NONE',  ( 5.700000000000002842, 2.725425358843983450E-16, -9.332722423957255486 ) ) ;
#16284=ORIENTED_EDGE ( 'NONE', *, *, #2179, .F. ) ;
#16297=CARTESIAN_POINT ( 'NONE',  ( -3.814044456245444081, 4.235925505221192822, -12.00000000000000533 ) ) ;
#16299=CARTESIAN_POINT ( 'NONE',  ( 1.761396867937200073, 5.421022142882376826, -13.31249999590322730 ) ) ;
#16307=CIRCLE ( 'NONE', #13749, 5.700000000000001954 ) ;
#16312=EDGE_LOOP ( 'NONE', ( #16949, #9494, #16760, #10829 ) ) ;
#16319=ORIENTED_EDGE ( 'NONE', *, *, #790, .F. ) ;
#16322=CARTESIAN_POINT ( 'NONE',  ( 3.954556930911861112, 2.873153789725825913, -14.84374999795161543 ) ) ;
#16323=CARTESIAN_POINT ( 'NONE',  ( -4.080749450109650844, 4.080749450109650844, -9.812499995903225525 ) ) ;
#16326=CARTESIAN_POINT ( 'NONE',  ( -4.620319390059841602, -1.773574444220693325, -11.96874999795161365 ) ) ;
#16328=ORIENTED_EDGE ( 'NONE', *, *, #13163, .T. ) ;
#16332=CARTESIAN_POINT ( 'NONE',  ( 3.954556930911842016, -2.873153789725853002, -8.843749997951615427 ) ) ;
#16334=CARTESIAN_POINT ( 'NONE',  ( 4.465502636338025688, -1.988169868018592856, -14.84374999795161543 ) ) ;
#16351=VERTEX_POINT ( 'NONE', #2919 ) ;
#16363=FACE_OUTER_BOUND ( 'NONE', #8520, .T. ) ;
#16364=MANIFOLD_SOLID_BREP ( 'Thread1', #16073 ) ;
#16366=CARTESIAN_POINT ( 'NONE',  ( 3.143139765844623401, 4.840010801796480244, -9.500000000000003553 ) ) ;
#16374=CARTESIAN_POINT ( 'NONE',  ( -5.700000000000000178, -2.180340287075187351E-16, -13.97977757194593273 ) ) ;
#16400=CARTESIAN_POINT ( 'NONE',  ( 4.780397808154265960, 1.280903732194420996, -8.968749997951613651 ) ) ;
#16415=CARTESIAN_POINT ( 'NONE',  ( 4.233219804643871598, -2.444050593750019651, -11.84374999795161365 ) ) ;
#16419=( GEOMETRIC_REPRESENTATION_CONTEXT ( 3 ) GLOBAL_UNCERTAINTY_ASSIGNED_CONTEXT ( ( #6780 ) ) GLOBAL_UNIT_ASSIGNED_CONTEXT ( ( #9507, #18794, #1794 ) ) REPRESENTATION_CONTEXT ( 'NONE', 'WORKASPACE' ) );
#16436=CARTESIAN_POINT ( 'NONE',  ( 2.620002426024508502, -5.142044285764769462, -10.81249999590322375 ) ) ;
#16438=ORIENTED_EDGE ( 'NONE', *, *, #4503, .T. ) ;
#16453=AXIS2_PLACEMENT_3D ( 'NONE', #16171, #14757, #19539 ) ;
#16458=VECTOR ( 'NONE', #6572, 1000.000000000000000 ) ;
#16459=EDGE_CURVE ( 'NONE', #3194, #768, #645, .T. ) ;
#16460=ORIENTED_EDGE ( 'NONE', *, *, #13746, .F. ) ;
#16470=CARTESIAN_POINT ( 'NONE',  ( -4.942249507334558700, -0.2590123213420631454, -12.96874999795161543 ) ) ;
#16471=CARTESIAN_POINT ( 'NONE',  ( -0.5958122406256771697, -5.668774803599153422, -9.312499995903225525 ) ) ;
#16473=EDGE_LOOP ( 'NONE', ( #5093, #14123, #10933, #16225, #17635 ) ) ;
#16474=DIRECTION ( 'NONE',  ( 0.000000000000000000, 0.000000000000000000, 1.000000000000000000 ) ) ;
#16485=ORIENTED_EDGE ( 'NONE', *, *, #10679, .T. ) ;
#16498=CARTESIAN_POINT ( 'NONE',  ( -2.444050593749990341, 4.233219804643887585, -6.468749997951615427 ) ) ;
#16499=CARTESIAN_POINT ( 'NONE',  ( -3.631840208645857437, -4.484949146646330931, -7.812499995903224637 ) ) ;
#16503=CARTESIAN_POINT ( 'NONE',  ( -2.444050593750049849, -4.233219804643852946, -6.468749997951615427 ) ) ;
#16528=CARTESIAN_POINT ( 'NONE',  ( -4.781284448697201483, -1.016293382781378485, -12.46874999795161543 ) ) ;
#16535=CARTESIAN_POINT ( 'NONE',  ( 3.499494075959815653, 3.499494075959816541, -14.34374999795161365 ) ) ;
#16546=SURFACE_STYLE_FILL_AREA ( #17946 ) ;
#16552=CARTESIAN_POINT ( 'NONE',  ( 2.850000000000024070, 4.936344801571289409, -7.312499995903225525 ) ) ;
#16570=CARTESIAN_POINT ( 'NONE',  ( 0.5958122406256382009, 5.668774803599156975, -8.000000000000005329 ) ) ;
#16575=CARTESIAN_POINT ( 'NONE',  ( -1.773574444220725521, 4.620319390059830056, -7.343749997951615427 ) ) ;
#16578=CARTESIAN_POINT ( 'NONE',  ( 2.318398865532074193, 5.207209108562820710, -9.000000000000005329 ) ) ;
#16596=CARTESIAN_POINT ( 'NONE',  ( 3.114526743279282694, 3.846120219227923798, -6.968749997951614539 ) ) ;
#16601=CARTESIAN_POINT ( 'NONE',  ( -4.781284448697179279, 1.016293382781477961, -10.46874999795161720 ) ) ;
#16603=ORIENTED_EDGE ( 'NONE', *, *, #13662, .T. ) ;
#16605=CARTESIAN_POINT ( 'NONE',  ( -5.668774803599153422, 0.5958122406256767256, -14.31249999590322552 ) ) ;
#16609=FACE_OUTER_BOUND ( 'NONE', #18828, .T. ) ;
#16619=VECTOR ( 'NONE', #16024, 1000.000000000000000 ) ;
#16625=CARTESIAN_POINT ( 'NONE',  ( -2.993098736590125853E-16, 4.888101187500000222, -11.46874999795161543 ) ) ;
#16637=ORIENTED_EDGE ( 'NONE', *, *, #16064, .F. ) ;
#16657=CARTESIAN_POINT ( 'NONE',  ( 4.861323657744411442, 0.5109457054261445919, -9.468749997951615427 ) ) ;
#16667=CARTESIAN_POINT ( 'NONE',  ( -3.143139765844656264, -4.840010801796461593, -10.81249999590322375 ) ) ;
#16671=LINE ( 'NONE', #14679, #15619 ) ;
#16681=EDGE_CURVE ( 'NONE', #5756, #4658, #11791, .T. ) ;
#16711=VERTEX_POINT ( 'NONE', #19709 ) ;
#16724=AXIS2_PLACEMENT_3D ( 'NONE', #17428, #9833, #6230 ) ;
#16728=CARTESIAN_POINT ( 'NONE',  ( -3.846120219227966430, -3.114526743279228072, -10.96874999795161720 ) ) ;
#16738=CARTESIAN_POINT ( 'NONE',  ( -3.499494075959816541, 3.499494075959816541, -8.968749997951613651 ) ) ;
#16758=ADVANCED_FACE ( 'NONE', ( #1308 ), #7386, .F. ) ;
#16759=( BOUNDED_CURVE ( )  B_SPLINE_CURVE ( 2, ( #8609, #19021, #14718, #5312, #13304, #19406, #11809, #17912, #4204, #10320, #16415, #2692, #15212, #9210, #1504, #7281, #12207 ),
 .UNSPECIFIED., .F., .F. ) 
 B_SPLINE_CURVE_WITH_KNOTS ( ( 3, 2, 2, 2, 2, 2, 2, 2, 3 ),
 ( 0.000000000000000000, 0.05000000000000000971, 0.1000000000000000194, 0.1499999999999999944, 0.2000000000000000389, 0.2500000000000000000, 0.2999999999999999889, 0.3499999999999999223, 0.4000000000000000777 ),
 .UNSPECIFIED. ) 
 CURVE ( )  GEOMETRIC_REPRESENTATION_ITEM ( )  RATIONAL_B_SPLINE_CURVE ( ( 1.000000000000000000, 0.9876883405951377704, 1.000000000000000000, 0.9876883405951377704, 1.000000000000000000, 0.9876883405951377704, 1.000000000000000000, 0.9876883405951377704, 1.000000000000000000, 0.9876883405951377704, 1.000000000000000000, 0.9876883405951377704, 1.000000000000000000, 0.9876883405951377704, 1.000000000000000000, 0.9876883405951377704, 1.000000000000000000 ) ) 
 REPRESENTATION_ITEM ( '' )  );
#16760=ORIENTED_EDGE ( 'NONE', *, *, #19203, .F. ) ;
#16768=EDGE_CURVE ( 'NONE', #8931, #6178, #9754, .T. ) ;
#16773=FACE_OUTER_BOUND ( 'NONE', #16473, .T. ) ;
#16775=ORIENTED_EDGE ( 'NONE', *, *, #17146, .F. ) ;
#16778=CARTESIAN_POINT ( 'NONE',  ( 5.574407415329156734, -1.493657965219523209, -14.81249999590322552 ) ) ;
#16783=DIRECTION ( 'NONE',  ( -0.000000000000000000, -0.000000000000000000, 1.000000000000000000 ) ) ;
#16806=CARTESIAN_POINT ( 'NONE',  ( 2.850000000000024070, 4.936344801571289409, -6.656249997951614539 ) ) ;
#16810=DIRECTION ( 'NONE',  ( -0.000000000000000000, -0.000000000000000000, 1.000000000000000000 ) ) ;
#16811=ADVANCED_FACE ( 'NONE', ( #3889 ), #13827, .T. ) ;
#16817=ORIENTED_EDGE ( 'NONE', *, *, #13612, .T. ) ;
#16823=CARTESIAN_POINT ( 'NONE',  ( 5.207209108562820710, -2.318398865532073305, -14.00000000000000533 ) ) ;
#16829=CARTESIAN_POINT ( 'NONE',  ( 4.942249507334556924, 0.2590123213420975623, -13.34374999795161365 ) ) ;
#16850=FACE_OUTER_BOUND ( 'NONE', #18610, .T. ) ;
#16864=CARTESIAN_POINT ( 'NONE',  ( -2.444050593749990341, 4.233219804643887585, -6.468749997951615427 ) ) ;
#16879=VECTOR ( 'NONE', #14893, 1000.000000000000000 ) ;
#16898=CARTESIAN_POINT ( 'NONE',  ( -5.699999999999999289, 0.9027913098498568933, -6.500000000000005329 ) ) ;
#16905=CARTESIAN_POINT ( 'NONE',  ( 0.000000000000000000, 0.000000000000000000, -22.00000000000000000 ) ) ;
#16906=CARTESIAN_POINT ( 'NONE',  ( 0.000000000000000000, 0.000000000000000000, -28.99999999999999645 ) ) ;
#16908=CARTESIAN_POINT ( 'NONE',  ( -2.850000000000058265, -4.936344801571268093, -7.312499995903225525 ) ) ;
#16915=ORIENTED_EDGE ( 'NONE', *, *, #1660, .F. ) ;
#16920=EDGE_CURVE ( 'NONE', #4658, #12853, #2875, .T. ) ;
#16921=CARTESIAN_POINT ( 'NONE',  ( 2.444050593749960587, -4.233219804643904460, -6.468749997951615427 ) ) ;
#16933=CARTESIAN_POINT ( 'NONE',  ( 2.246813503491833508, 4.409619785863906571, -13.34374999795161365 ) ) ;
#16934=CARTESIAN_POINT ( 'NONE',  ( 2.246813503491803310, -4.409619785863921670, -10.34374999795161543 ) ) ;
#16946=DIRECTION ( 'NONE',  ( -0.8090169943749481174, -0.5877852522924720269, 0.000000000000000000 ) ) ;
#16949=ORIENTED_EDGE ( 'NONE', *, *, #18082, .F. ) ;
#16960=ORIENTED_EDGE ( 'NONE', *, *, #13305, .T. ) ;
#16971=CARTESIAN_POINT ( 'NONE',  ( 3.846120219227944670, 3.114526743279256493, -11.34374999795161543 ) ) ;
#16990=CARTESIAN_POINT ( 'NONE',  ( -5.668774803599153422, 0.5958122406256767256, -14.31249999590322552 ) ) ;
#16994=CARTESIAN_POINT ( 'NONE',  ( -4.648860486681953397, 1.510506337161861445, -7.468749997951615427 ) ) ;
#17018=CARTESIAN_POINT ( 'NONE',  ( -4.611396867937224364, -3.350375938067065906, -14.00000000000000533 ) ) ;
#17041=CARTESIAN_POINT ( 'NONE',  ( -4.861323657744403448, 0.5109457054262118714, -13.84374999795161543 ) ) ;
#17042=CARTESIAN_POINT ( 'NONE',  ( 3.632567103900546712, 3.270778111535313837, -7.468749997951615427 ) ) ;
#17044=CARTESIAN_POINT ( 'NONE',  ( 2.695436003842704764, -4.150607464521812062, -12.96874999795161543 ) ) ;
#17045=EDGE_CURVE ( 'NONE', #19526, #4220, #2831, .T. ) ;
#17046=VERTEX_POINT ( 'NONE', #16498 ) ;
#17051=STYLED_ITEM ( 'NONE', ( #2086 ), #9489 ) ;
#17053=EDGE_CURVE ( 'NONE', #8931, #736, #2774, .T. ) ;
#17059=VECTOR ( 'NONE', #13111, 1000.000000000000000 ) ;
#17064=CARTESIAN_POINT ( 'NONE',  ( -3.814044456245531567, -4.235925505221111997, -10.00000000000000533 ) ) ;
#17072=CARTESIAN_POINT ( 'NONE',  ( 0.000000000000000000, 0.000000000000000000, -6.000000000000005329 ) ) ;
#17076=CARTESIAN_POINT ( 'NONE',  ( -5.700000000000000178, -2.180340287075187351E-16, -12.66727757604271076 ) ) ;
#17079=VERTEX_POINT ( 'NONE', #6171 ) ;
#17091=CARTESIAN_POINT ( 'NONE',  ( -4.465502636338051445, -1.988169868018530462, -8.843749997951615427 ) ) ;
#17100=DIRECTION ( 'NONE',  ( -0.4330127018922284576, -0.7499999999999961142, 0.4999999999999977240 ) ) ;
#17101=CARTESIAN_POINT ( 'NONE',  ( 1.510506337161829027, -4.648860486681964055, -10.46874999795161720 ) ) ;
#17103=AXIS2_PLACEMENT_3D ( 'NONE', #16905, #16810, #4981 ) ;
#17111=CARTESIAN_POINT ( 'NONE',  ( 5.700000000000001954, -0.5990941410143687529, -9.668198987696284163 ) ) ;
#17138=EDGE_CURVE ( 'NONE', #17079, #5861, #4885, .T. ) ;
#17139=CARTESIAN_POINT ( 'NONE',  ( -4.235925505221191933, -3.814044456245443193, -7.000000000000005329 ) ) ;
#17141=ORIENTED_EDGE ( 'NONE', *, *, #17053, .T. ) ;
#17145=ORIENTED_EDGE ( 'NONE', *, *, #15895, .F. ) ;
#17146=EDGE_CURVE ( 'NONE', #3827, #9061, #10982, .T. ) ;
#17160=CARTESIAN_POINT ( 'NONE',  ( -5.668774803599153422, 0.5958122406256767256, -13.00000000000000533 ) ) ;
#17175=CARTESIAN_POINT ( 'NONE',  ( 2.849999999999954348, -4.936344801571327601, -6.000000000000005329 ) ) ;
#17180=CARTESIAN_POINT ( 'NONE',  ( 9.000000000000000000, 0.000000000000000000, -28.99999999999999645 ) ) ;
#17181=ORIENTED_EDGE ( 'NONE', *, *, #15518, .T. ) ;
#17186=CARTESIAN_POINT ( 'NONE',  ( -1.510506337161861667, 4.648860486681953397, -10.46874999795161720 ) ) ;
#17197=CARTESIAN_POINT ( 'NONE',  ( 0.9027913098498173694, -5.700000000000005507, -10.50000000000000711 ) ) ;
#17201=SURFACE_STYLE_FILL_AREA ( #15698 ) ;
#17210=DIRECTION ( 'NONE',  ( -0.4330127018922234616, -0.7499999999999990008, 0.4999999999999978351 ) ) ;
#17231=CARTESIAN_POINT ( 'NONE',  ( 0.5958122406255995651, -5.668774803599162304, -15.31249999590322552 ) ) ;
#17240=EDGE_LOOP ( 'NONE', ( #2494, #18240, #13864, #13902 ) ) ;
#17245=EDGE_CURVE ( 'NONE', #17330, #12027, #19748, .T. ) ;
#17263=VECTOR ( 'NONE', #11992, 1000.000000000000000 ) ;
#17265=CARTESIAN_POINT ( 'NONE',  ( -4.781284448697179279, 1.016293382781477961, -10.84374999795161543 ) ) ;
#17295=CARTESIAN_POINT ( 'NONE',  ( 5.700000000000001066, -3.980288726281172656E-14, -6.000000000000005329 ) ) ;
#17302=AXIS2_PLACEMENT_3D ( 'NONE', #13844, #15448, #7728 ) ;
#17307=ORIENTED_EDGE ( 'NONE', *, *, #10527, .T. ) ;
#17308=FACE_OUTER_BOUND ( 'NONE', #7309, .T. ) ;
#17323=CARTESIAN_POINT ( 'NONE',  ( -5.575441324182679459, 1.185096637661293251, -11.31249999590322375 ) ) ;
#17327=LINE ( 'NONE', #8519, #14061 ) ;
#17330=VERTEX_POINT ( 'NONE', #5493 ) ;
#17346=CARTESIAN_POINT ( 'NONE',  ( -4.233219804643904460, -2.444050593749961031, -11.46874999795161543 ) ) ;
#17353=DIRECTION ( 'NONE',  ( 1.000000000000000000, 0.000000000000000000, 0.000000000000000000 ) ) ;
#17369=VERTEX_POINT ( 'NONE', #15918 ) ;
#17378=CARTESIAN_POINT ( 'NONE',  ( 1.280903732194454303, 4.780397808154257078, -8.968749997951611874 ) ) ;
#17393=ADVANCED_FACE ( 'NONE', ( #2201 ), #13210, .T. ) ;
#17405=CARTESIAN_POINT ( 'NONE',  ( 5.294050593750000644, -3.696815770993907903E-14, -7.078124996927420476 ) ) ;
#17408=CARTESIAN_POINT ( 'NONE',  ( 4.936344801571289409, -2.850000000000023626, -12.31249999590322552 ) ) ;
#17413=CARTESIAN_POINT ( 'NONE',  ( 2.444050593749960587, -4.233219804643904460, -6.843749997951615427 ) ) ;
#17426=VERTEX_POINT ( 'NONE', #12915 ) ;
#17428=CARTESIAN_POINT ( 'NONE',  ( 0.000000000000000000, 0.000000000000000000, 0.000000000000000000 ) ) ;
#17432=ORIENTED_EDGE ( 'NONE', *, *, #15895, .T. ) ;
#17439=CARTESIAN_POINT ( 'NONE',  ( 1.988169868018562880, -4.465502636338038123, -13.84374999795161543 ) ) ;
#17442=FACE_OUTER_BOUND ( 'NONE', #7073, .T. ) ;
#17463=CARTESIAN_POINT ( 'NONE',  ( 0.000000000000000000, 0.000000000000000000, 0.000000000000000000 ) ) ;
#17472=EDGE_CURVE ( 'NONE', #5267, #1462, #6913, .T. ) ;
#17473=CARTESIAN_POINT ( 'NONE',  ( -4.465502636338051445, -1.988169868018530462, -8.843749997951615427 ) ) ;
#17477=CARTESIAN_POINT ( 'NONE',  ( -0.2590123213420971182, 4.942249507334556924, -7.968749997951616315 ) ) ;
#17480=ORIENTED_EDGE ( 'NONE', *, *, #8714, .T. ) ;
#17481=CARTESIAN_POINT ( 'NONE',  ( -4.861323657744413218, -0.5109457054261099529, -9.468749997951615427 ) ) ;
#17487=AXIS2_PLACEMENT_3D ( 'NONE', #15482, #18971, #8638 ) ;
#17495=CARTESIAN_POINT ( 'NONE',  ( 3.350375938067065462, -4.611396867937225252, -9.000000000000005329 ) ) ;
#17521=CARTESIAN_POINT ( 'NONE',  ( 4.611396867937200383, 3.350375938067097881, -14.00000000000000533 ) ) ;
#17529=CARTESIAN_POINT ( 'NONE',  ( -2.850000000000058265, -4.936344801571268093, -6.656249997951614539 ) ) ;
#17538=CARTESIAN_POINT ( 'NONE',  ( 1.016293382781377819, -4.781284448697200595, -7.843749997951614539 ) ) ;
#17545=CARTESIAN_POINT ( 'NONE',  ( 3.499494075959791672, -3.499494075959840966, -9.343749997951615427 ) ) ;
#17550=CARTESIAN_POINT ( 'NONE',  ( 3.954556930911842016, -2.873153789725853002, -8.468749997951615427 ) ) ;
#17560=CARTESIAN_POINT ( 'NONE',  ( 2.246813503491803310, -4.409619785863921670, -10.34374999795161543 ) ) ;
#17573=CARTESIAN_POINT ( 'NONE',  ( -3.270778111535288080, 3.632567103900569361, -12.46874999795161543 ) ) ;
#17577=CARTESIAN_POINT ( 'NONE',  ( -3.631840208645857437, -4.484949146646330931, -6.500000000000005329 ) ) ;
#17604=CARTESIAN_POINT ( 'NONE',  ( -4.780397808154247308, 1.280903732194486722, -14.34374999795161543 ) ) ;
#17616=EDGE_LOOP ( 'NONE', ( #12435, #13609, #8045, #12826 ) ) ;
#17629=DIRECTION ( 'NONE',  ( -1.000000000000000000, 0.000000000000000000, 0.000000000000000000 ) ) ;
#17635=ORIENTED_EDGE ( 'NONE', *, *, #353, .F. ) ;
#17644=CARTESIAN_POINT ( 'NONE',  ( -3.954556930911881096, -2.873153789725797935, -14.46874999795161720 ) ) ;
#17655=EDGE_CURVE ( 'NONE', #9505, #8042, #3214, .T. ) ;
#17656=CARTESIAN_POINT ( 'NONE',  ( 0.7741991708318548548, -4.888101187500005551, -10.96874999795161720 ) ) ;
#17663=CARTESIAN_POINT ( 'NONE',  ( 4.888101187500000222, -3.413342815706642518E-14, -6.843749997951615427 ) ) ;
#17671=ORIENTED_EDGE ( 'NONE', *, *, #7191, .T. ) ;
#17672=CARTESIAN_POINT ( 'NONE',  ( -4.780397808154273953, -1.280903732194386579, -9.343749997951615427 ) ) ;
#17697=CARTESIAN_POINT ( 'NONE',  ( 4.150607464521812062, 2.695436003842704764, -8.343749997951611874 ) ) ;
#17701=CARTESIAN_POINT ( 'NONE',  ( 2.873153789725825025, 3.954556930911862000, -13.84374999795161543 ) ) ;
#17718=DIRECTION ( 'NONE',  ( -0.000000000000000000, -0.000000000000000000, 1.000000000000000000 ) ) ;
#17727=CARTESIAN_POINT ( 'NONE',  ( 3.350375938067096548, 4.611396867937201272, -13.00000000000000533 ) ) ;
#17748=CARTESIAN_POINT ( 'NONE',  ( -4.465502636338010589, 1.988169868018623720, -14.46874999795161720 ) ) ;
#17763=CARTESIAN_POINT ( 'NONE',  ( -4.200000000000001954, 5.143516556418886872E-16, -6.000000000000005329 ) ) ;
#17798=CARTESIAN_POINT ( 'NONE',  ( 1.988169868018562880, -4.465502636338038123, -13.46874999795161543 ) ) ;
#17800=CARTESIAN_POINT ( 'NONE',  ( -4.465502636338010589, 1.988169868018623720, -14.84374999795161543 ) ) ;
#17827=CARTESIAN_POINT ( 'NONE',  ( -0.5109457054262123155, -4.861323657744403448, -8.843749997951615427 ) ) ;
#17832=CARTESIAN_POINT ( 'NONE',  ( 3.350375938067065462, -4.611396867937225252, -10.31249999590322552 ) ) ;
#17834=CARTESIAN_POINT ( 'NONE',  ( 4.781284448697194378, 1.016293382781411792, -12.46874999795161543 ) ) ;
#17846=DIRECTION ( 'NONE',  ( -0.000000000000000000, -0.000000000000000000, 1.000000000000000000 ) ) ;
#17866=CARTESIAN_POINT ( 'NONE',  ( 1.773574444220693103, -4.620319390059841602, -6.968749997951614539 ) ) ;
#17871=FACE_OUTER_BOUND ( 'NONE', #2261, .T. ) ;
#17879=ORIENTED_EDGE ( 'NONE', *, *, #2082, .T. ) ;
#17887=CYLINDRICAL_SURFACE ( 'NONE', #13970, 4.200000000000001066 ) ;
#17896=CARTESIAN_POINT ( 'NONE',  ( 3.632567103900546712, 3.270778111535313837, -7.468749997951615427 ) ) ;
#17902=AXIS2_PLACEMENT_3D ( 'NONE', #18120, #15317, #15706 ) ;
#17906=VECTOR ( 'NONE', #2142, 1000.000000000000114 ) ;
#17910=DIRECTION ( 'NONE',  ( -0.000000000000000000, -0.000000000000000000, 1.000000000000000000 ) ) ;
#17912=CARTESIAN_POINT ( 'NONE',  ( 4.942249507334556036, -0.2590123213421313686, -10.34374999795161543 ) ) ;
#17913=CARTESIAN_POINT ( 'NONE',  ( -0.5109457054261112852, 4.861323657744413218, -14.84374999795161543 ) ) ;
#17915=( BOUNDED_SURFACE ( )  B_SPLINE_SURFACE ( 1, 2, ( 
 ( #18004, #16499, #8893, #1288, #7365, #13487, #18097, #2877, #4387, #1393, #9493, #4977, #14079, #15786, #1971, #3381, #18485 ),
 ( #9393, #18391, #12685, #4881, #17091, #18583, #4781, #10788, #6359, #83, #3477, #4684, #13988, #15684, #1686, #15393, #3570 ) ),
 .UNSPECIFIED., .F., .F., .F. ) 
 B_SPLINE_SURFACE_WITH_KNOTS ( ( 2, 2 ),
 ( 3, 2, 2, 2, 2, 2, 2, 2, 3 ),
 ( 0.000000000000000000, 1.000000000000000000 ),
 ( 0.000000000000000000, 0.05000000000000000278, 0.1000000000000000056, 0.1499999999999999944, 0.2000000000000000111, 0.2500000000000000000, 0.2999999999999999889, 0.3499999999999999778, 0.4000000000000000222 ),
 .UNSPECIFIED. ) 
 GEOMETRIC_REPRESENTATION_ITEM ( )  RATIONAL_B_SPLINE_SURFACE ( (
 ( 1.000000000000000000, 0.9876883405951377704, 1.000000000000000000, 0.9876883405951377704, 1.000000000000000000, 0.9876883405951377704, 1.000000000000000000, 0.9876883405951377704, 1.000000000000000000, 0.9876883405951377704, 1.000000000000000000, 0.9876883405951377704, 1.000000000000000000, 0.9876883405951377704, 1.000000000000000000, 0.9876883405951377704, 1.000000000000000000),
 ( 1.000000000000000000, 0.9876883405951377704, 1.000000000000000000, 0.9876883405951377704, 1.000000000000000000, 0.9876883405951377704, 1.000000000000000000, 0.9876883405951377704, 1.000000000000000000, 0.9876883405951377704, 1.000000000000000000, 0.9876883405951377704, 1.000000000000000000, 0.9876883405951377704, 1.000000000000000000, 0.9876883405951377704, 1.000000000000000000) ) ) 
 REPRESENTATION_ITEM ( '' )  SURFACE ( )  );
#17925=CARTESIAN_POINT ( 'NONE',  ( -2.620002426024544473, 5.142044285764750811, -9.500000000000005329 ) ) ;
#17927=CARTESIAN_POINT ( 'NONE',  ( -1.280903732194487166, -4.780397808154247308, -8.968749997951611874 ) ) ;
#17929=ADVANCED_FACE ( 'NONE', ( #4539 ), #13750, .F. ) ;
#17934=CYLINDRICAL_SURFACE ( 'NONE', #1016, 5.700000000000001954 ) ;
#17935=CARTESIAN_POINT ( 'NONE',  ( 5.699999999999994849, -0.9027913098498965283, -7.812499995903224637 ) ) ;
#17946=FILL_AREA_STYLE ('',( #5723 ) ) ;
#17965=CONICAL_SURFACE ( 'NONE', #8367, 9.000000000000001776, 0.6898000447336081198 ) ;
#17969=ORIENTED_EDGE ( 'NONE', *, *, #15579, .T. ) ;
#17970=CARTESIAN_POINT ( 'NONE',  ( -3.270778111535363131, -3.632567103900500971, -10.46874999795161720 ) ) ;
#17980=CARTESIAN_POINT ( 'NONE',  ( 5.575441324182695446, 1.185096637661215757, -12.00000000000000533 ) ) ;
#18004=CARTESIAN_POINT ( 'NONE',  ( -2.850000000000058265, -4.936344801571268093, -7.312499995903225525 ) ) ;
#18042=CARTESIAN_POINT ( 'NONE',  ( 3.270778111535338262, 3.632567103900523620, -10.84374999795161543 ) ) ;
#18051=DIRECTION ( 'NONE',  ( 0.8660254037844398178, -6.047423072554923456E-15, 0.4999999999999979461 ) ) ;
#18052=CARTESIAN_POINT ( 'NONE',  ( -2.246813503491864150, -4.409619785863891472, -12.96874999795161543 ) ) ;
#18060=DIRECTION ( 'NONE',  ( -0.000000000000000000, -0.000000000000000000, 1.000000000000000000 ) ) ;
#18063=CARTESIAN_POINT ( 'NONE',  ( 0.5109457054261454800, -4.861323657744410554, -14.46874999795161720 ) ) ;
#18066=CARTESIAN_POINT ( 'NONE',  ( -0.2590123213420971182, 4.942249507334556924, -7.968749997951616315 ) ) ;
#18068=CARTESIAN_POINT ( 'NONE',  ( -4.465502636338010589, 1.988169868018623720, -14.46874999795161720 ) ) ;
#18070=ORIENTED_EDGE ( 'NONE', *, *, #17138, .F. ) ;
#18082=EDGE_CURVE ( 'NONE', #5861, #6550, #8630, .T. ) ;
#18086=VECTOR ( 'NONE', #12428, 1000.000000000000000 ) ;
#18096=CARTESIAN_POINT ( 'NONE',  ( 4.861323657744411442, 0.5109457054261445919, -9.468749997951615427 ) ) ;
#18097=CARTESIAN_POINT ( 'NONE',  ( -5.668774803599165857, -0.5958122406255588199, -10.31249999590322552 ) ) ;
#18120=CARTESIAN_POINT ( 'NONE',  ( 0.000000000000000000, 0.000000000000000000, 0.000000000000000000 ) ) ;
#18124=CARTESIAN_POINT ( 'NONE',  ( 4.780397808154257078, -1.280903732194453637, -14.34374999795161543 ) ) ;
#18129=ORIENTED_EDGE ( 'NONE', *, *, #9622, .F. ) ;
#18133=CARTESIAN_POINT ( 'NONE',  ( 3.954556930911861112, 2.873153789725825913, -14.84374999795161543 ) ) ;
#18134=CARTESIAN_POINT ( 'NONE',  ( 1.510506337161829027, -4.648860486681964055, -10.84374999795161543 ) ) ;
#18152=ORIENTED_EDGE ( 'NONE', *, *, #134, .F. ) ;
#18168=CARTESIAN_POINT ( 'NONE',  ( 4.861323657744406113, -0.5109457054261780096, -13.46874999795161543 ) ) ;
#18170=CARTESIAN_POINT ( 'NONE',  ( 5.574407415329156734, -1.493657965219523209, -13.50000000000000533 ) ) ;
#18175=CARTESIAN_POINT ( 'NONE',  ( 0.5958122406256377568, 5.668774803599156975, -9.312499995903225525 ) ) ;
#18181=CARTESIAN_POINT ( 'NONE',  ( 2.849999999999954348, -4.936344801571327601, -6.000000000000005329 ) ) ;
#18184=ADVANCED_FACE ( 'NONE', ( #8827 ), #17934, .T. ) ;
#18233=CARTESIAN_POINT ( 'NONE',  ( -0.7741991708318890497, 4.888101187500000222, -11.34374999795161543 ) ) ;
#18240=ORIENTED_EDGE ( 'NONE', *, *, #14888, .T. ) ;
#18244=EDGE_LOOP ( 'NONE', ( #1063, #17145, #8252, #18459 ) ) ;
#18246=DIRECTION ( 'NONE',  ( -0.000000000000000000, -0.000000000000000000, 1.000000000000000000 ) ) ;
#18258=CARTESIAN_POINT ( 'NONE',  ( 4.840010801796506890, 3.143139765844590983, -7.500000000000005329 ) ) ;
#18265=CONICAL_SURFACE ( 'NONE', #17302, 9.000000000000001776, 0.6898000447336081198 ) ;
#18267=CARTESIAN_POINT ( 'NONE',  ( -4.484949146646406426, -3.631840208645763735, -11.81249999590322552 ) ) ;
#18294=CARTESIAN_POINT ( 'NONE',  ( 5.207209108562820710, -2.318398865532073305, -15.31249999590322552 ) ) ;
#18303=AXIS2_PLACEMENT_3D ( 'NONE', #15672, #4668, #12471 ) ;
#18316=EDGE_CURVE ( 'NONE', #15854, #14057, #10726, .T. ) ;
#18321=CARTESIAN_POINT ( 'NONE',  ( 2.695436003842732298, 4.150607464521792522, -10.34374999795161543 ) ) ;
#18327=CARTESIAN_POINT ( 'NONE',  ( 1.510506337161861223, 4.648860486681953397, -12.46874999795161543 ) ) ;
#18346=DIRECTION ( 'NONE',  ( -0.9135454576425999784, 0.4067366430758019846, 0.000000000000000000 ) ) ;
#18359=CARTESIAN_POINT ( 'NONE',  ( 0.5109457054261784537, 4.861323657744407001, -8.468749997951615427 ) ) ;
#18369=CARTESIAN_POINT ( 'NONE',  ( 3.143139765844622957, 4.840010801796481132, -10.81249999590322375 ) ) ;
#18370=ORIENTED_EDGE ( 'NONE', *, *, #2179, .T. ) ;
#18372=ADVANCED_FACE ( 'NONE', ( #13624 ), #6676, .T. ) ;
#18376=PLANE ( 'NONE',  #18303 ) ;
#18378=CARTESIAN_POINT ( 'NONE',  ( -1.761396867937238042, -5.421022142882365280, -13.31249999590322730 ) ) ;
#18391=CARTESIAN_POINT ( 'NONE',  ( -3.114526743279308896, -3.846120219227901149, -7.343749997951615427 ) ) ;
#18415=CARTESIAN_POINT ( 'NONE',  ( -2.444050593749990785, 4.233219804643887585, -6.843749997951615427 ) ) ;
#18422=CARTESIAN_POINT ( 'NONE',  ( 3.499494075959815653, 3.499494075959816541, -13.96874999795161365 ) ) ;
#18429=ORIENTED_EDGE ( 'NONE', *, *, #163, .T. ) ;
#18441=( BOUNDED_CURVE ( )  B_SPLINE_CURVE ( 2, ( #8504, #18805, #513, #6581, #2001 ),
 .UNSPECIFIED., .F., .F. ) 
 B_SPLINE_CURVE_WITH_KNOTS ( ( 3, 2, 3 ),
 ( 0.3333180920165872418, 0.3499999999999999778, 0.4000000000000000222 ),
 .UNSPECIFIED. ) 
 CURVE ( )  GEOMETRIC_REPRESENTATION_ITEM ( )  RATIONAL_B_SPLINE_CURVE ( ( 0.9945256517182510247, 0.9958923606136993456, 1.000000000000000000, 0.9876883405951377704, 1.000000000000000000 ) ) 
 REPRESENTATION_ITEM ( '' )  );
#18445=EDGE_CURVE ( 'NONE', #19252, #3827, #15624, .T. ) ;
#18459=ORIENTED_EDGE ( 'NONE', *, *, #10114, .F. ) ;
#18462=CARTESIAN_POINT ( 'NONE',  ( 4.781284448697195266, 1.016293382781411792, -12.84374999795161543 ) ) ;
#18485=CARTESIAN_POINT ( 'NONE',  ( -0.5958122406255597081, 5.668774803599165857, -15.31249999590322552 ) ) ;
#18499=FILL_AREA_STYLE_COLOUR ( '', #8100 ) ;
#18505=CARTESIAN_POINT ( 'NONE',  ( 5.700000000000001066, -4.360680574150373717E-16, -12.66727757604273386 ) ) ;
#18507=CARTESIAN_POINT ( 'NONE',  ( 2.318398865532038666, -5.207209108562836697, -13.00000000000000533 ) ) ;
#18512=CARTESIAN_POINT ( 'NONE',  ( -2.873153789725825469, 3.954556930911862000, -9.843749997951615427 ) ) ;
#18530=CARTESIAN_POINT ( 'NONE',  ( -4.888101187500000222, 0.000000000000000000, -6.843749997951615427 ) ) ;
#18533=PLANE ( 'NONE',  #9177 ) ;
#18534=CARTESIAN_POINT ( 'NONE',  ( -2.850000000000058265, -4.936344801571268093, -6.000000000000005329 ) ) ;
#18578=CARTESIAN_POINT ( 'NONE',  ( -0.5958122406256771697, -5.668774803599153422, -9.312499995903225525 ) ) ;
#18583=CARTESIAN_POINT ( 'NONE',  ( -4.780397808154273953, -1.280903732194386579, -9.343749997951615427 ) ) ;
#18598=FACE_OUTER_BOUND ( 'NONE', #14631, .T. ) ;
#18602=DIRECTION ( 'NONE',  ( 0.000000000000000000, 0.000000000000000000, 1.000000000000000000 ) ) ;
#18609=CARTESIAN_POINT ( 'NONE',  ( -0.7741991708318890497, 4.888101187500000222, -11.34374999795161543 ) ) ;
#18610=EDGE_LOOP ( 'NONE', ( #5002, #6460, #10731, #5032, #15511 ) ) ;
#18626=DIRECTION ( 'NONE',  ( -0.6363829547955638377, 0.000000000000000000, -0.7713732785400770897 ) ) ;
#18628=CARTESIAN_POINT ( 'NONE',  ( 4.936344801571289409, -2.850000000000023626, -12.31249999590322552 ) ) ;
#18631=CARTESIAN_POINT ( 'NONE',  ( -4.465502636338010589, 1.988169868018623720, -14.84374999795161543 ) ) ;
#18661=CARTESIAN_POINT ( 'NONE',  ( -4.780397808154273953, -1.280903732194386579, -9.343749997951615427 ) ) ;
#18680=CARTESIAN_POINT ( 'NONE',  ( -0.7741991708318890497, 4.888101187500000222, -10.96874999795161720 ) ) ;
#18690=CARTESIAN_POINT ( 'NONE',  ( 0.7741991708318548548, -4.888101187500005551, -10.96874999795161720 ) ) ;
#18712=ADVANCED_FACE ( 'NONE', ( #2400 ), #14620, .F. ) ;
#18727=CARTESIAN_POINT ( 'NONE',  ( 1.016293382781377819, -4.781284448697200595, -7.843749997951614539 ) ) ;
#18738=AXIS2_PLACEMENT_3D ( 'NONE', #15302, #13491, #2880 ) ;
#18750=CARTESIAN_POINT ( 'NONE',  ( -5.574407415329146964, 1.493657965219562067, -13.50000000000000533 ) ) ;
#18768=EDGE_LOOP ( 'NONE', ( #16485, #17307, #11426, #14230 ) ) ;
#18774=CARTESIAN_POINT ( 'NONE',  ( -4.235925505221191933, -3.814044456245443193, -7.000000000000005329 ) ) ;
#18778=CARTESIAN_POINT ( 'NONE',  ( 0.7741991708318884946, 4.888101187500000222, -11.96874999795161365 ) ) ;
#18786=( BOUNDED_SURFACE ( )  B_SPLINE_SURFACE ( 1, 2, ( 
 ( #10277, #15070, #10671, #12370, #18175, #12072, #256, #18369, #2853, #15167, #3053, #7442, #7848, #1759, #4856, #16778, #7546 ),
 ( #12268, #16575, #15470, #4660, #13566, #4754, #9168, #6338, #15274, #16971, #13964, #10571, #18462, #3253, #12463, #13867, #159 ) ),
 .UNSPECIFIED., .F., .F., .F. ) 
 B_SPLINE_SURFACE_WITH_KNOTS ( ( 2, 2 ),
 ( 3, 2, 2, 2, 2, 2, 2, 2, 3 ),
 ( 0.000000000000000000, 1.000000000000000000 ),
 ( 0.000000000000000000, 0.05000000000000000278, 0.1000000000000000056, 0.1499999999999999944, 0.2000000000000000111, 0.2500000000000000000, 0.2999999999999999889, 0.3499999999999999778, 0.4000000000000000222 ),
 .UNSPECIFIED. ) 
 GEOMETRIC_REPRESENTATION_ITEM ( )  RATIONAL_B_SPLINE_SURFACE ( (
 ( 1.000000000000000000, 0.9876883405951377704, 1.000000000000000000, 0.9876883405951377704, 1.000000000000000000, 0.9876883405951377704, 1.000000000000000000, 0.9876883405951377704, 1.000000000000000000, 0.9876883405951377704, 1.000000000000000000, 0.9876883405951377704, 1.000000000000000000, 0.9876883405951377704, 1.000000000000000000, 0.9876883405951377704, 1.000000000000000000),
 ( 1.000000000000000000, 0.9876883405951377704, 1.000000000000000000, 0.9876883405951377704, 1.000000000000000000, 0.9876883405951377704, 1.000000000000000000, 0.9876883405951377704, 1.000000000000000000, 0.9876883405951377704, 1.000000000000000000, 0.9876883405951377704, 1.000000000000000000, 0.9876883405951377704, 1.000000000000000000, 0.9876883405951377704, 1.000000000000000000) ) ) 
 REPRESENTATION_ITEM ( '' )  SURFACE ( )  );
#18789=CARTESIAN_POINT ( 'NONE',  ( -4.235925505221191933, -3.814044456245443193, -8.312499995903225525 ) ) ;
#18794=( NAMED_UNIT ( * ) PLANE_ANGLE_UNIT ( ) SI_UNIT ( $, .RADIAN. ) );
#18796=CARTESIAN_POINT ( 'NONE',  ( 4.484949146646379781, 3.631840208645794821, -11.81249999590322552 ) ) ;
#18798=FACE_OUTER_BOUND ( 'NONE', #14555, .T. ) ;
#18805=CARTESIAN_POINT ( 'NONE',  ( 5.700000000000001066, -0.2987243419133421840, -14.14705514798869679 ) ) ;
#18807=EDGE_CURVE ( 'NONE', #8919, #15015, #11549, .T. ) ;
#18811=AXIS2_PLACEMENT_3D ( 'NONE', #15142, #18246, #13639 ) ;
#18819=CARTESIAN_POINT ( 'NONE',  ( -0.5958122406255597081, 5.668774803599165857, -15.31249999590322552 ) ) ;
#18828=EDGE_LOOP ( 'NONE', ( #12453, #5136, #13406, #7972 ) ) ;
#18832=AXIS2_PLACEMENT_3D ( 'NONE', #14561, #12957, #13053 ) ;
#18842=CARTESIAN_POINT ( 'NONE',  ( -4.861323657744403448, 0.5109457054262118714, -13.46874999795161543 ) ) ;
#18845=DIRECTION ( 'NONE',  ( -0.000000000000000000, -0.000000000000000000, 1.000000000000000000 ) ) ;
#18879=CARTESIAN_POINT ( 'NONE',  ( -1.280903732194386802, 4.780397808154273065, -13.96874999795161365 ) ) ;
#18899=CARTESIAN_POINT ( 'NONE',  ( 5.574407415329170057, 1.493657965219485018, -9.812499995903223748 ) ) ;
#18928=FACE_OUTER_BOUND ( 'NONE', #13257, .T. ) ;
#18932=ORIENTED_EDGE ( 'NONE', *, *, #6801, .F. ) ;
#18945=CARTESIAN_POINT ( 'NONE',  ( 4.080749450109622423, -4.080749450109678378, -8.500000000000005329 ) ) ;
#18950=EDGE_LOOP ( 'NONE', ( #4643, #14299, #9466, #17480, #10091 ) ) ;
#18956=CARTESIAN_POINT ( 'NONE',  ( 4.409619785863891472, -2.246813503491864150, -8.343749997951611874 ) ) ;
#18968=CARTESIAN_POINT ( 'NONE',  ( -4.781284448697179279, 1.016293382781477961, -10.46874999795161720 ) ) ;
#18971=DIRECTION ( 'NONE',  ( -0.000000000000000000, -0.000000000000000000, 1.000000000000000000 ) ) ;
#18993=CARTESIAN_POINT ( 'NONE',  ( -2.246813503491864150, -4.409619785863891472, -12.96874999795161543 ) ) ;
#18997=CARTESIAN_POINT ( 'NONE',  ( 5.700000000000001066, 0.5990941410143484358, -13.64430100820693603 ) ) ;
#18998=ORIENTED_EDGE ( 'NONE', *, *, #15621, .T. ) ;
#19006=DIRECTION ( 'NONE',  ( 0.1045284632676418274, -0.9945218953682745111, 0.000000000000000000 ) ) ;
#19007=CARTESIAN_POINT ( 'NONE',  ( -5.142044285764750811, 2.620002426024544029, -8.812499995903225525 ) ) ;
#19020=CARTESIAN_POINT ( 'NONE',  ( -5.387740456496205255, 2.068159791354258648, -11.81249999590322552 ) ) ;
#19021=CARTESIAN_POINT ( 'NONE',  ( 3.114526743279282694, 3.846120219227923798, -7.343749997951615427 ) ) ;
#19032=CARTESIAN_POINT ( 'NONE',  ( -5.700000000000000178, 0.9027913098498568933, -6.500000000000005329 ) ) ;
#19045=CARTESIAN_POINT ( 'NONE',  ( 0.7741991708318548548, -4.888101187500005551, -10.96874999795161720 ) ) ;
#19055=CARTESIAN_POINT ( 'NONE',  ( 3.954556930911842016, -2.873153789725853002, -8.843749997951615427 ) ) ;
#19056=DIRECTION ( 'NONE',  ( -0.000000000000000000, -0.000000000000000000, 1.000000000000000000 ) ) ;
#19065=CARTESIAN_POINT ( 'NONE',  ( -4.465502636338051445, -1.988169868018530462, -8.468749997951615427 ) ) ;
#19067=CARTESIAN_POINT ( 'NONE',  ( 4.942249507334556924, 0.2590123213420971182, -12.96874999795161543 ) ) ;
#19082=DIRECTION ( 'NONE',  ( 1.000000000000000000, 0.000000000000000000, 0.000000000000000000 ) ) ;
#19099=CARTESIAN_POINT ( 'NONE',  ( 4.080749450109649956, 4.080749450109650844, -14.81249999590322552 ) ) ;
#19128=CARTESIAN_POINT ( 'NONE',  ( 0.9027913098498565603, 5.700000000000000178, -11.50000000000000355 ) ) ;
#19138=EDGE_LOOP ( 'NONE', ( #4294, #3068, #11408, #18152 ) ) ;
#19152=FACE_OUTER_BOUND ( 'NONE', #1808, .T. ) ;
#19160=CARTESIAN_POINT ( 'NONE',  ( -5.700000000000001066, 1.090170143537592985E-15, -9.332722423957234170 ) ) ;
#19172=CARTESIAN_POINT ( 'NONE',  ( 0.5958122406256382009, 5.668774803599156975, -8.000000000000005329 ) ) ;
#19194=CARTESIAN_POINT ( 'NONE',  ( -1.988169868018624609, -4.465502636338009701, -9.843749997951615427 ) ) ;
#19197=CARTESIAN_POINT ( 'NONE',  ( 2.850000000000024070, 4.936344801571289409, -7.312499995903225525 ) ) ;
#19203=EDGE_CURVE ( 'NONE', #4244, #1462, #7055, .T. ) ;
#19217=DIRECTION ( 'NONE',  ( 0.000000000000000000, 0.000000000000000000, -1.000000000000000000 ) ) ;
#19230=CARTESIAN_POINT ( 'NONE',  ( 4.648860486681943627, -1.510506337161893864, -7.843749997951614539 ) ) ;
#19233=CARTESIAN_POINT ( 'NONE',  ( -2.620002426024580000, -5.142044285764733935, -12.50000000000000533 ) ) ;
#19244=CARTESIAN_POINT ( 'NONE',  ( 4.648860486681943627, -1.510506337161893864, -7.468749997951615427 ) ) ;
#19252=VERTEX_POINT ( 'NONE', #4469 ) ;
#19258=CARTESIAN_POINT ( 'NONE',  ( -2.444050593750049849, -4.233219804643852946, -6.843749997951615427 ) ) ;
#19282=DIRECTION ( 'NONE',  ( 0.000000000000000000, 0.000000000000000000, -1.000000000000000000 ) ) ;
#19317=CARTESIAN_POINT ( 'NONE',  ( -4.781284448697201483, -1.016293382781378485, -12.84374999795161543 ) ) ;
#19323=B_SPLINE_CURVE_WITH_KNOTS ( 'NONE', 1,
 ( #9650, #6615 ),
 .UNSPECIFIED., .F., .F.,
 ( 2, 2 ),
 ( 0.000000000000000000, 1.000000000000000000 ),
 .UNSPECIFIED. ) ;
#19325=CARTESIAN_POINT ( 'NONE',  ( 5.700000000000001066, -3.980288726281172656E-14, -7.312499995903225525 ) ) ;
#19328=CARTESIAN_POINT ( 'NONE',  ( -3.350375938067128967, -4.611396867937178179, -13.00000000000000533 ) ) ;
#19331=LINE ( 'NONE', #15855, #17906 ) ;
#19337=CARTESIAN_POINT ( 'NONE',  ( 0.5745956068257360716, -5.466912017135475033, -14.11718749948790830 ) ) ;
#19344=PLANE ( 'NONE',  #16453 ) ;
#19349=AXIS2_PLACEMENT_3D ( 'NONE', #5855, #19464, #11972 ) ;
#19355=CARTESIAN_POINT ( 'NONE',  ( -1.988169868018530906, 4.465502636338051445, -13.46874999795161543 ) ) ;
#19357=CARTESIAN_POINT ( 'NONE',  ( 3.814044456245502701, 4.235925505221138643, -10.00000000000000533 ) ) ;
#19358=VERTEX_POINT ( 'NONE', #9378 ) ;
#19361=ADVANCED_FACE ( 'NONE', ( #168 ), #18376, .F. ) ;
#19367=CARTESIAN_POINT ( 'NONE',  ( 4.936344801571308061, 2.849999999999989431, -11.00000000000000711 ) ) ;
#19386=CARTESIAN_POINT ( 'NONE',  ( -0.5958122406255597081, 5.668774803599165857, -14.00000000000000533 ) ) ;
#19390=CARTESIAN_POINT ( 'NONE',  ( -3.490243377569957047E-16, 5.700000000000001066, -12.31249999590322552 ) ) ;
#19406=CARTESIAN_POINT ( 'NONE',  ( 4.780397808154265960, 1.280903732194420996, -9.343749997951615427 ) ) ;
#19425=CARTESIAN_POINT ( 'NONE',  ( -3.945386292505473391E-14, -5.700000000000001066, -12.31249999590322552 ) ) ;
#19426=( BOUNDED_CURVE ( )  B_SPLINE_CURVE ( 2, ( #12030, #12331, #6008, #4512, #10629, #3116, #3014, #16934, #18134, #8828, #13418, #9025, #14931, #4322, #8925, #1320, #13724 ),
 .UNSPECIFIED., .F., .F. ) 
 B_SPLINE_CURVE_WITH_KNOTS ( ( 3, 2, 2, 2, 2, 2, 2, 2, 3 ),
 ( 0.000000000000000000, 0.05000000000000000971, 0.1000000000000000194, 0.1499999999999999944, 0.2000000000000000389, 0.2500000000000000000, 0.2999999999999999889, 0.3499999999999999223, 0.4000000000000000777 ),
 .UNSPECIFIED. ) 
 CURVE ( )  GEOMETRIC_REPRESENTATION_ITEM ( )  RATIONAL_B_SPLINE_CURVE ( ( 1.000000000000000000, 0.9876883405951377704, 1.000000000000000000, 0.9876883405951377704, 1.000000000000000000, 0.9876883405951377704, 1.000000000000000000, 0.9876883405951377704, 1.000000000000000000, 0.9876883405951377704, 1.000000000000000000, 0.9876883405951377704, 1.000000000000000000, 0.9876883405951377704, 1.000000000000000000, 0.9876883405951377704, 1.000000000000000000 ) ) 
 REPRESENTATION_ITEM ( '' )  );
#19428=CARTESIAN_POINT ( 'NONE',  ( 4.942249507334556924, 0.2590123213420971182, -12.96874999795161543 ) ) ;
#19443=LINE ( 'NONE', #11557, #15176 ) ;
#19445=CIRCLE ( 'NONE', #18811, 5.700000000000001954 ) ;
#19464=DIRECTION ( 'NONE',  ( -0.4067366430758074247, -0.9135454576425977580, 0.000000000000000000 ) ) ;
#19486=CARTESIAN_POINT ( 'NONE',  ( -2.993098736590125853E-16, 4.888101187500000222, -11.84374999795161365 ) ) ;
#19506=AXIS2_PLACEMENT_3D ( 'NONE', #19337, #8641, #14748 ) ;
#19517=AXIS2_PLACEMENT_3D ( 'NONE', #757, #17846, #13337 ) ;
#19518=CARTESIAN_POINT ( 'NONE',  ( -0.7741991708318890497, 4.888101187500000222, -10.96874999795161720 ) ) ;
#19521=CARTESIAN_POINT ( 'NONE',  ( 5.574407415329170057, 1.493657965219485018, -8.500000000000005329 ) ) ;
#19526=VERTEX_POINT ( 'NONE', #19160 ) ;
#19531=CARTESIAN_POINT ( 'NONE',  ( -2.246813503491864150, -4.409619785863891472, -13.34374999795161365 ) ) ;
#19539=DIRECTION ( 'NONE',  ( -1.000000000000000000, 0.000000000000000000, -0.000000000000000000 ) ) ;
#19544=AXIS2_PLACEMENT_3D ( 'NONE', #909, #6988, #13110 ) ;
#19547=CARTESIAN_POINT ( 'NONE',  ( 5.574407415329170057, 1.493657965219485018, -8.500000000000007105 ) ) ;
#19551=CARTESIAN_POINT ( 'NONE',  ( 4.780397808154257078, -1.280903732194453859, -13.96874999795161365 ) ) ;
#19553=CARTESIAN_POINT ( 'NONE',  ( -4.781284448697201483, -1.016293382781378485, -12.46874999795161543 ) ) ;
#19555=CIRCLE ( 'NONE', #6767, 4.200000000000000178 ) ;
#19556=VERTEX_POINT ( 'NONE', #17763 ) ;
#19611=CARTESIAN_POINT ( 'NONE',  ( 0.5958122406255995651, -5.668774803599162304, -15.31249999590322552 ) ) ;
#19618=CARTESIAN_POINT ( 'NONE',  ( -1.016293382781411569, 4.781284448697194378, -7.843749997951614539 ) ) ;
#19626=CARTESIAN_POINT ( 'NONE',  ( -3.499494075959816541, 3.499494075959816541, -9.343749997951615427 ) ) ;
#19641=CARTESIAN_POINT ( 'NONE',  ( -3.499494075959840078, -3.499494075959791672, -13.96874999795161365 ) ) ;
#19656=CARTESIAN_POINT ( 'NONE',  ( 3.814044456245474279, -4.235925505221167064, -12.00000000000000533 ) ) ;
#19661=CARTESIAN_POINT ( 'NONE',  ( 1.016293382781377819, -4.781284448697200595, -7.468749997951615427 ) ) ;
#19672=DIRECTION ( 'NONE',  ( 1.000000000000000000, 0.000000000000000000, 0.000000000000000000 ) ) ;
#19693=CARTESIAN_POINT ( 'NONE',  ( -2.695436003842674122, 4.150607464521828938, -12.96874999795161543 ) ) ;
#19706=CARTESIAN_POINT ( 'NONE',  ( 0.5958122406255970116, -5.668774803599162304, 0.000000000000000000 ) ) ;
#19709=CARTESIAN_POINT ( 'NONE',  ( -0.5109457054261112852, 4.861323657744413218, -14.46874999795161720 ) ) ;
#19716=ORIENTED_EDGE ( 'NONE', *, *, #9672, .T. ) ;
#19717=CARTESIAN_POINT ( 'NONE',  ( -4.620319390059841602, -1.773574444220693325, -12.34374999795161543 ) ) ;
#19719=ORIENTED_EDGE ( 'NONE', *, *, #443, .F. ) ;
#19723=CARTESIAN_POINT ( 'NONE',  ( -4.888101187500000222, 0.000000000000000000, -6.843749997951615427 ) ) ;
#19724=ORIENTED_EDGE ( 'NONE', *, *, #14674, .T. ) ;
#19725=CARTESIAN_POINT ( 'NONE',  ( -1.773574444220725077, 4.620319390059829168, -7.343749997951615427 ) ) ;
#19726=EDGE_CURVE ( 'NONE', #15015, #5395, #3885, .T. ) ;
#19727=CARTESIAN_POINT ( 'NONE',  ( -4.409619785863906571, 2.246813503491833508, -7.968749997951616315 ) ) ;
#19730=ORIENTED_EDGE ( 'NONE', *, *, #12598, .T. ) ;
#19731=FACE_OUTER_BOUND ( 'NONE', #4773, .T. ) ;
#19746=VECTOR ( 'NONE', #16474, 1000.000000000000000 ) ;
#19748=LINE ( 'NONE', #8755, #9950 ) ;
#19749=CARTESIAN_POINT ( 'NONE',  ( 1.493657965219485462, -5.574407415329169169, -13.50000000000000533 ) ) ;
#19751=ORIENTED_EDGE ( 'NONE', *, *, #2082, .F. ) ;
#19752=CARTESIAN_POINT ( 'NONE',  ( 3.270778111535338262, 3.632567103900523620, -10.46874999795161720 ) ) ;
#19754=DIRECTION ( 'NONE',  ( -0.4999999999999920619, 0.8660254037844432595, 0.000000000000000000 ) ) ;
#19770=CARTESIAN_POINT ( 'NONE',  ( 2.620002426024508502, -5.142044285764769462, -10.81249999590322375 ) ) ;
ENDSEC;
END-ISO-10303-21;
